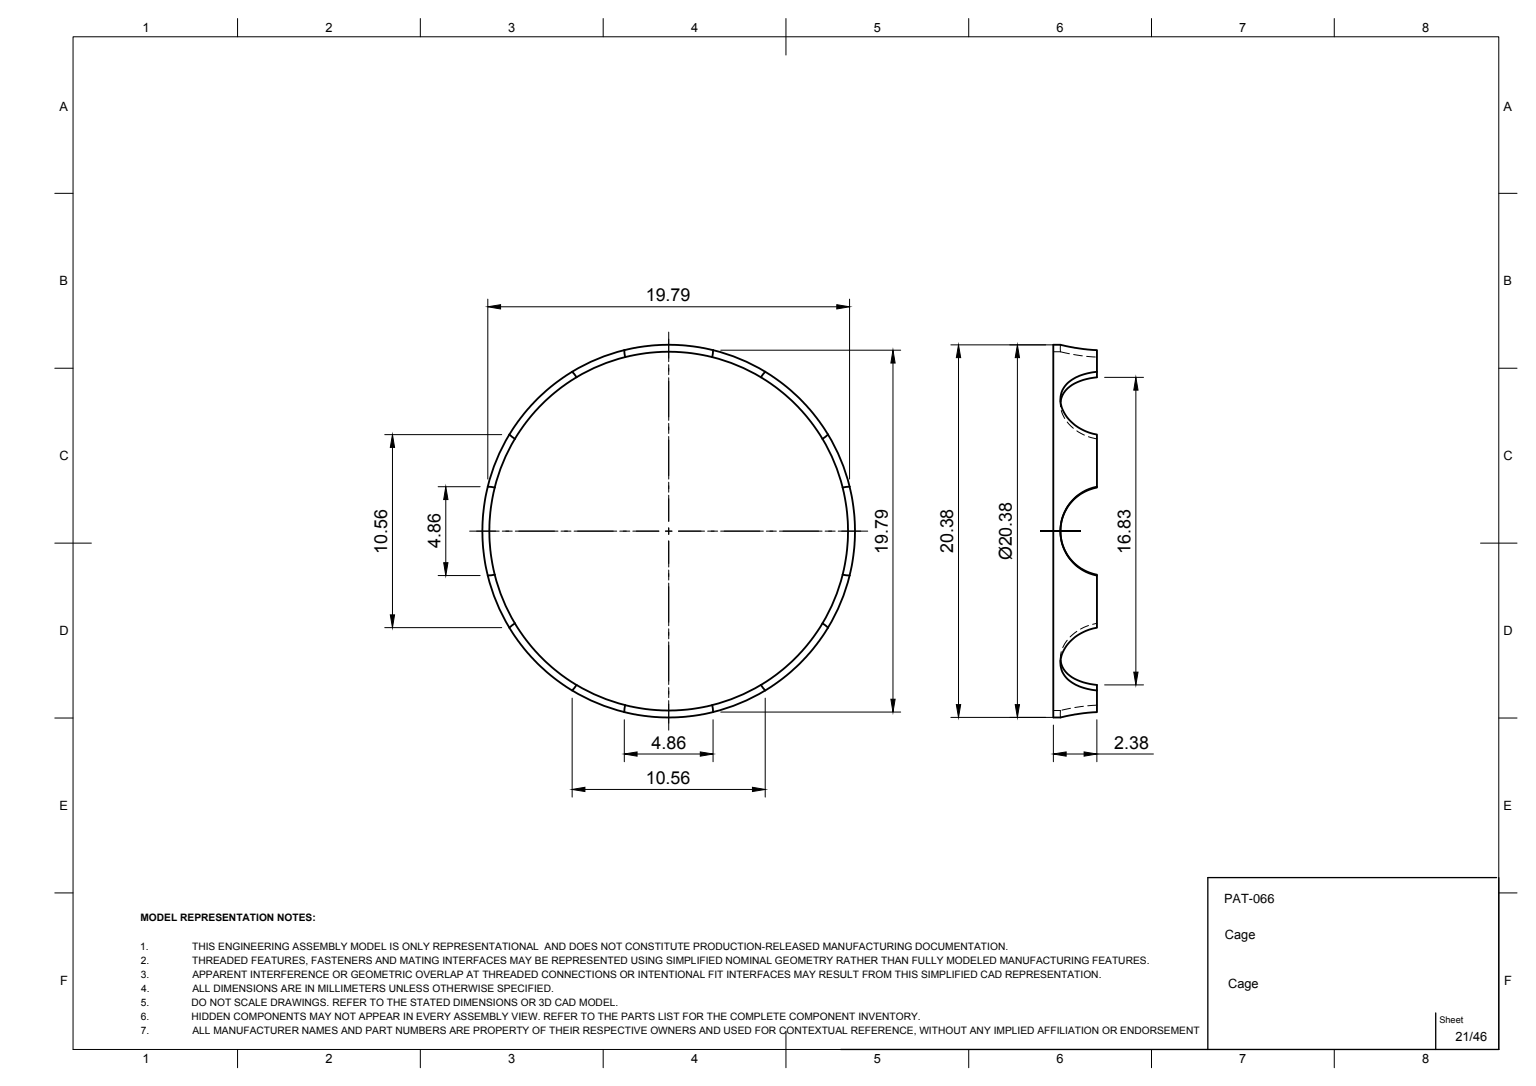
ISO-10303-21;
HEADER;
/* Generated by software containing ST-Developer
 * from STEP Tools, Inc. (www.steptools.com) 
 */

FILE_DESCRIPTION(
/* description */ ('Lever-operated bar clamp (toggle)'),
/* implementation_level */ '2;1');

FILE_NAME(
/* name */ 'Cage.step',
/* time_stamp */ '2026-10-28T03:25:02-07:00',
/* author */ (''),
/* organization */ (''),
/* preprocessor_version */ 'ST-DEVELOPER v20.2',
/* originating_system */ 'Autodesk Translation Framework v15.17.0.0',
/* authorisation */ '');

FILE_SCHEMA (('AUTOMOTIVE_DESIGN { 1 0 10303 214 3 1 1 }'));
ENDSEC;

DATA;
#10=MECHANICAL_DESIGN_GEOMETRIC_PRESENTATION_REPRESENTATION('',(#432),#12413);
#263=B_SPLINE_CURVE_WITH_KNOTS('',3,(#10837,#10838,#10839,#10840,#10841,
#10842,#10843,#10844,#10845,#10846,#10847,#10848,#10849,#10850,#10851,#10852,
#10853,#10854,#10855,#10856,#10857,#10858),.UNSPECIFIED.,.F.,.F.,(4,2,2,
2,2,2,2,2,2,2,4),(0.0473477652366656,0.126350602536658,0.189525903804987,
0.252701205073317,0.313298422430275,0.373895639787233,0.434492857144191,
0.495090074501149,0.558265375769478,0.621440677037807,0.7004435143378),
 .UNSPECIFIED.);
#264=B_SPLINE_CURVE_WITH_KNOTS('',3,(#10862,#10863,#10864,#10865,#10866,
#10867,#10868,#10869,#10870,#10871,#10872,#10873,#10874,#10875,#10876,#10877,
#10878,#10879,#10880,#10881,#10882,#10883),.UNSPECIFIED.,.F.,.F.,(4,2,2,
2,2,2,2,2,2,2,4),(0.0464897534940957,0.0852567806515119,0.170513561303024,
0.246687263103517,0.308657850341199,0.370628437578881,0.432599024816563,
0.494569612054245,0.570743313854739,0.656000094506251,0.694767121663666),
 .UNSPECIFIED.);
#265=B_SPLINE_CURVE_WITH_KNOTS('',3,(#10889,#10890,#10891,#10892,#10893,
#10894,#10895,#10896,#10897,#10898,#10899,#10900,#10901,#10902,#10903,#10904,
#10905,#10906,#10907,#10908,#10909,#10910),.UNSPECIFIED.,.F.,.F.,(4,2,2,
2,2,2,2,2,2,2,4),(0.0464897534940957,0.0852567806515118,0.170513561303024,
0.246687263103517,0.308657850341199,0.370628437578881,0.432599024816563,
0.494569612054245,0.570743313854738,0.65600009450625,0.694767121663666),
 .UNSPECIFIED.);
#266=B_SPLINE_CURVE_WITH_KNOTS('',3,(#10914,#10915,#10916,#10917,#10918,
#10919,#10920,#10921,#10922,#10923,#10924,#10925,#10926,#10927,#10928,#10929,
#10930,#10931,#10932,#10933,#10934,#10935),.UNSPECIFIED.,.F.,.F.,(4,2,2,
2,2,2,2,2,2,2,4),(0.0464897534940957,0.0852567806515119,0.170513561303024,
0.246687263103517,0.308657850341199,0.370628437578881,0.432599024816563,
0.494569612054245,0.570743313854739,0.656000094506251,0.694767121663666),
 .UNSPECIFIED.);
#267=B_SPLINE_CURVE_WITH_KNOTS('',3,(#10939,#10940,#10941,#10942,#10943,
#10944,#10945,#10946,#10947,#10948,#10949,#10950),.UNSPECIFIED.,.F.,.F.,
(4,2,2,2,2,4),(0.0464897534940957,0.0852567806515119,0.170513561303024,
0.246687263103517,0.308657850341199,0.370628437578881),.UNSPECIFIED.);
#268=B_SPLINE_CURVE_WITH_KNOTS('',3,(#10955,#10956,#10957,#10958,#10959,
#10960,#10961,#10962,#10963,#10964,#10965,#10966),.UNSPECIFIED.,.F.,.F.,
(4,2,2,2,2,4),(0.370628437578881,0.432599024816563,0.494569612054245,0.570743313854738,
0.65600009450625,0.694767121663666),.UNSPECIFIED.);
#269=B_SPLINE_CURVE_WITH_KNOTS('',3,(#10970,#10971,#10972,#10973,#10974,
#10975,#10976,#10977,#10978,#10979,#10980,#10981,#10982,#10983,#10984,#10985,
#10986,#10987,#10988,#10989,#10990,#10991),.UNSPECIFIED.,.F.,.F.,(4,2,2,
2,2,2,2,2,2,2,4),(0.0464897534940957,0.0852567806515121,0.170513561303024,
0.246687263103518,0.308657850341199,0.370628437578881,0.432599024816563,
0.494569612054245,0.570743313854738,0.65600009450625,0.694767121663666),
 .UNSPECIFIED.);
#270=B_SPLINE_CURVE_WITH_KNOTS('',3,(#10995,#10996,#10997,#10998,#10999,
#11000,#11001,#11002,#11003,#11004,#11005,#11006,#11007,#11008,#11009,#11010,
#11011,#11012,#11013,#11014,#11015,#11016),.UNSPECIFIED.,.F.,.F.,(4,2,2,
2,2,2,2,2,2,2,4),(0.0464897534940957,0.0852567806515119,0.170513561303024,
0.246687263103517,0.308657850341199,0.370628437578881,0.432599024816563,
0.494569612054245,0.570743313854738,0.65600009450625,0.694767121663667),
 .UNSPECIFIED.);
#271=B_SPLINE_CURVE_WITH_KNOTS('',3,(#11020,#11021,#11022,#11023,#11024,
#11025,#11026,#11027,#11028,#11029,#11030,#11031,#11032,#11033,#11034,#11035,
#11036,#11037,#11038,#11039,#11040,#11041),.UNSPECIFIED.,.F.,.F.,(4,2,2,
2,2,2,2,2,2,2,4),(0.0464897534940957,0.0852567806515119,0.170513561303024,
0.246687263103517,0.308657850341199,0.370628437578881,0.432599024816563,
0.494569612054245,0.570743313854738,0.65600009450625,0.694767121663666),
 .UNSPECIFIED.);
#272=B_SPLINE_CURVE_WITH_KNOTS('',3,(#11045,#11046,#11047,#11048,#11049,
#11050,#11051,#11052,#11053,#11054,#11055,#11056,#11057,#11058,#11059,#11060,
#11061,#11062,#11063,#11064,#11065,#11066),.UNSPECIFIED.,.F.,.F.,(4,2,2,
2,2,2,2,2,2,2,4),(0.0464897534940957,0.0852567806515119,0.170513561303024,
0.246687263103517,0.308657850341199,0.370628437578881,0.432599024816563,
0.494569612054245,0.570743313854739,0.656000094506251,0.694767121663667),
 .UNSPECIFIED.);
#273=B_SPLINE_CURVE_WITH_KNOTS('',3,(#11074,#11075,#11076,#11077,#11078,
#11079,#11080,#11081,#11082,#11083,#11084,#11085,#11086,#11087,#11088,#11089,
#11090,#11091,#11092,#11093,#11094,#11095),.UNSPECIFIED.,.F.,.F.,(4,2,2,
2,2,2,2,2,2,2,4),(0.0473477652366656,0.126350602536658,0.189525903804987,
0.252701205073316,0.313298422430274,0.373895639787232,0.434492857144191,
0.495090074501149,0.558265375769478,0.621440677037807,0.7004435143378),
 .UNSPECIFIED.);
#274=B_SPLINE_CURVE_WITH_KNOTS('',3,(#11103,#11104,#11105,#11106,#11107,
#11108,#11109,#11110,#11111,#11112,#11113,#11114,#11115,#11116,#11117,#11118,
#11119,#11120,#11121,#11122,#11123,#11124),.UNSPECIFIED.,.F.,.F.,(4,2,2,
2,2,2,2,2,2,2,4),(0.0473477652366656,0.126350602536658,0.189525903804987,
0.252701205073317,0.313298422430275,0.373895639787233,0.434492857144191,
0.495090074501149,0.558265375769478,0.621440677037807,0.7004435143378),
 .UNSPECIFIED.);
#275=B_SPLINE_CURVE_WITH_KNOTS('',3,(#11133,#11134,#11135,#11136,#11137,
#11138,#11139,#11140,#11141,#11142,#11143,#11144),.UNSPECIFIED.,.F.,.F.,
(4,2,2,2,2,4),(0.0473477652366656,0.126350602536658,0.189525903804987,0.252701205073316,
0.313298422430275,0.373895639787233),.UNSPECIFIED.);
#276=B_SPLINE_CURVE_WITH_KNOTS('',3,(#11146,#11147,#11148,#11149,#11150,
#11151,#11152,#11153,#11154,#11155,#11156,#11157),.UNSPECIFIED.,.F.,.F.,
(4,2,2,2,2,4),(0.373895639787233,0.434492857144191,0.495090074501149,0.558265375769478,
0.621440677037807,0.7004435143378),.UNSPECIFIED.);
#277=B_SPLINE_CURVE_WITH_KNOTS('',3,(#11164,#11165,#11166,#11167,#11168,
#11169,#11170,#11171,#11172,#11173,#11174,#11175,#11176,#11177,#11178,#11179,
#11180,#11181,#11182,#11183,#11184,#11185),.UNSPECIFIED.,.F.,.F.,(4,2,2,
2,2,2,2,2,2,2,4),(0.0473477652366656,0.126350602536658,0.189525903804987,
0.252701205073316,0.313298422430275,0.373895639787233,0.434492857144191,
0.495090074501149,0.558265375769478,0.621440677037807,0.7004435143378),
 .UNSPECIFIED.);
#278=B_SPLINE_CURVE_WITH_KNOTS('',3,(#11193,#11194,#11195,#11196,#11197,
#11198,#11199,#11200,#11201,#11202,#11203,#11204,#11205,#11206,#11207,#11208,
#11209,#11210,#11211,#11212,#11213,#11214),.UNSPECIFIED.,.F.,.F.,(4,2,2,
2,2,2,2,2,2,2,4),(0.0473477652366656,0.126350602536658,0.189525903804987,
0.252701205073317,0.313298422430275,0.373895639787233,0.434492857144191,
0.495090074501149,0.558265375769478,0.621440677037807,0.7004435143378),
 .UNSPECIFIED.);
#279=B_SPLINE_CURVE_WITH_KNOTS('',3,(#11222,#11223,#11224,#11225,#11226,
#11227,#11228,#11229,#11230,#11231,#11232,#11233,#11234,#11235,#11236,#11237,
#11238,#11239,#11240,#11241,#11242,#11243),.UNSPECIFIED.,.F.,.F.,(4,2,2,
2,2,2,2,2,2,2,4),(0.0473477652366656,0.126350602536658,0.189525903804987,
0.252701205073316,0.313298422430275,0.373895639787233,0.434492857144191,
0.495090074501149,0.558265375769478,0.621440677037807,0.7004435143378),
 .UNSPECIFIED.);
#280=B_SPLINE_CURVE_WITH_KNOTS('',3,(#11252,#11253,#11254,#11255,#11256,
#11257,#11258,#11259,#11260,#11261,#11262,#11263,#11264,#11265,#11266,#11267,
#11268,#11269,#11270,#11271,#11272,#11273),.UNSPECIFIED.,.F.,.F.,(4,2,2,
2,2,2,2,2,2,2,4),(0.0473477652366656,0.126350602536658,0.189525903804987,
0.252701205073317,0.313298422430275,0.373895639787233,0.434492857144191,
0.495090074501149,0.558265375769478,0.621440677037807,0.7004435143378),
 .UNSPECIFIED.);
#295=SPHERICAL_SURFACE('',#7386,0.247676);
#296=SPHERICAL_SURFACE('',#7402,0.247676);
#297=SPHERICAL_SURFACE('',#7407,0.247676);
#298=SPHERICAL_SURFACE('',#7412,0.247676);
#299=SPHERICAL_SURFACE('',#7417,0.247676);
#300=SPHERICAL_SURFACE('',#7422,0.247676);
#301=SPHERICAL_SURFACE('',#7427,0.247676);
#302=SPHERICAL_SURFACE('',#7435,0.247676);
#349=SHAPE_REPRESENTATION_RELATIONSHIP('SRR','None',#12589,#387);
#387=ADVANCED_BREP_SHAPE_REPRESENTATION('',(#478),#12386);
#432=STYLED_ITEM('',(#12869),#478);
#478=MANIFOLD_SOLID_BREP('Continuous crown cage',#6592);
#592=FACE_BOUND('',#1579,.T.);
#743=PLANE('',#7399);
#744=PLANE('',#7404);
#745=PLANE('',#7409);
#746=PLANE('',#7414);
#747=PLANE('',#7419);
#748=PLANE('',#7424);
#749=PLANE('',#7433);
#750=PLANE('',#7437);
#751=PLANE('',#7438);
#1063=FACE_OUTER_BOUND('',#1561,.T.);
#1064=FACE_OUTER_BOUND('',#1562,.T.);
#1065=FACE_OUTER_BOUND('',#1563,.T.);
#1066=FACE_OUTER_BOUND('',#1564,.T.);
#1067=FACE_OUTER_BOUND('',#1565,.T.);
#1068=FACE_OUTER_BOUND('',#1566,.T.);
#1069=FACE_OUTER_BOUND('',#1567,.T.);
#1070=FACE_OUTER_BOUND('',#1568,.T.);
#1071=FACE_OUTER_BOUND('',#1569,.T.);
#1072=FACE_OUTER_BOUND('',#1570,.T.);
#1073=FACE_OUTER_BOUND('',#1571,.T.);
#1074=FACE_OUTER_BOUND('',#1572,.T.);
#1075=FACE_OUTER_BOUND('',#1573,.T.);
#1076=FACE_OUTER_BOUND('',#1574,.T.);
#1077=FACE_OUTER_BOUND('',#1575,.T.);
#1078=FACE_OUTER_BOUND('',#1576,.T.);
#1079=FACE_OUTER_BOUND('',#1577,.T.);
#1080=FACE_OUTER_BOUND('',#1578,.T.);
#1081=FACE_OUTER_BOUND('',#1580,.T.);
#1561=EDGE_LOOP('',(#5125,#5126,#5127,#5128));
#1562=EDGE_LOOP('',(#5129,#5130,#5131,#5132,#5133,#5134,#5135,#5136,#5137,
#5138,#5139,#5140,#5141,#5142,#5143,#5144,#5145,#5146,#5147,#5148));
#1563=EDGE_LOOP('',(#5149,#5150,#5151,#5152));
#1564=EDGE_LOOP('',(#5153,#5154,#5155,#5156));
#1565=EDGE_LOOP('',(#5157,#5158,#5159,#5160));
#1566=EDGE_LOOP('',(#5161,#5162,#5163,#5164));
#1567=EDGE_LOOP('',(#5165,#5166,#5167,#5168));
#1568=EDGE_LOOP('',(#5169,#5170,#5171,#5172,#5173,#5174));
#1569=EDGE_LOOP('',(#5175,#5176,#5177,#5178));
#1570=EDGE_LOOP('',(#5179,#5180,#5181,#5182));
#1571=EDGE_LOOP('',(#5183,#5184,#5185,#5186));
#1572=EDGE_LOOP('',(#5187,#5188,#5189,#5190));
#1573=EDGE_LOOP('',(#5191,#5192,#5193,#5194));
#1574=EDGE_LOOP('',(#5195,#5196,#5197,#5198));
#1575=EDGE_LOOP('',(#5199,#5200,#5201,#5202,#5203,#5204,#5205,#5206,#5207,
#5208,#5209,#5210,#5211,#5212,#5213,#5214,#5215,#5216,#5217,#5218));
#1576=EDGE_LOOP('',(#5219,#5220,#5221,#5222));
#1577=EDGE_LOOP('',(#5223,#5224,#5225,#5226));
#1578=EDGE_LOOP('',(#5227));
#1579=EDGE_LOOP('',(#5228));
#1580=EDGE_LOOP('',(#5229,#5230,#5231,#5232));
#2050=LINE('',#10952,#2491);
#2051=LINE('',#11248,#2492);
#2491=VECTOR('',#8801,1.019052);
#2492=VECTOR('',#8878,0.980948);
#2886=CIRCLE('',#7387,0.243053047864041);
#2887=CIRCLE('',#7388,0.243053047864041);
#2888=CIRCLE('',#7390,1.019052);
#2889=CIRCLE('',#7391,1.019052);
#2890=CIRCLE('',#7392,1.019052);
#2891=CIRCLE('',#7393,1.019052);
#2892=CIRCLE('',#7394,1.019052);
#2893=CIRCLE('',#7395,1.019052);
#2894=CIRCLE('',#7396,1.019052);
#2895=CIRCLE('',#7397,1.019052);
#2896=CIRCLE('',#7398,1.019052);
#2897=CIRCLE('',#7400,0.980948);
#2898=CIRCLE('',#7401,0.243053047864041);
#2899=CIRCLE('',#7403,0.243053047864041);
#2900=CIRCLE('',#7405,0.980948);
#2901=CIRCLE('',#7406,0.243053047864041);
#2902=CIRCLE('',#7408,0.243053047864041);
#2903=CIRCLE('',#7410,0.980948);
#2904=CIRCLE('',#7411,0.243053047864041);
#2905=CIRCLE('',#7413,0.243053047864041);
#2906=CIRCLE('',#7415,0.980948);
#2907=CIRCLE('',#7416,0.243053047864041);
#2908=CIRCLE('',#7418,0.243053047864041);
#2909=CIRCLE('',#7420,0.980948);
#2910=CIRCLE('',#7421,0.243053047864041);
#2911=CIRCLE('',#7423,0.243053047864041);
#2912=CIRCLE('',#7425,0.980948);
#2913=CIRCLE('',#7426,0.243053047864041);
#2914=CIRCLE('',#7428,0.243053047864041);
#2915=CIRCLE('',#7430,0.980948);
#2916=CIRCLE('',#7431,0.980948);
#2917=CIRCLE('',#7432,0.980948);
#2918=CIRCLE('',#7434,0.243053047864041);
#2919=CIRCLE('',#7436,0.243053047864041);
#3317=VERTEX_POINT('',#10835);
#3318=VERTEX_POINT('',#10836);
#3319=VERTEX_POINT('',#10859);
#3320=VERTEX_POINT('',#10861);
#3321=VERTEX_POINT('',#10886);
#3322=VERTEX_POINT('',#10888);
#3323=VERTEX_POINT('',#10911);
#3324=VERTEX_POINT('',#10913);
#3325=VERTEX_POINT('',#10936);
#3326=VERTEX_POINT('',#10938);
#3327=VERTEX_POINT('',#10951);
#3328=VERTEX_POINT('',#10954);
#3329=VERTEX_POINT('',#10967);
#3330=VERTEX_POINT('',#10969);
#3331=VERTEX_POINT('',#10992);
#3332=VERTEX_POINT('',#10994);
#3333=VERTEX_POINT('',#11017);
#3334=VERTEX_POINT('',#11019);
#3335=VERTEX_POINT('',#11042);
#3336=VERTEX_POINT('',#11044);
#3337=VERTEX_POINT('',#11069);
#3338=VERTEX_POINT('',#11073);
#3339=VERTEX_POINT('',#11098);
#3340=VERTEX_POINT('',#11102);
#3341=VERTEX_POINT('',#11127);
#3342=VERTEX_POINT('',#11131);
#3343=VERTEX_POINT('',#11132);
#3344=VERTEX_POINT('',#11159);
#3345=VERTEX_POINT('',#11163);
#3346=VERTEX_POINT('',#11188);
#3347=VERTEX_POINT('',#11192);
#3348=VERTEX_POINT('',#11217);
#3349=VERTEX_POINT('',#11221);
#3350=VERTEX_POINT('',#11246);
#3351=VERTEX_POINT('',#11249);
#3352=VERTEX_POINT('',#11251);
#3967=EDGE_CURVE('',#3317,#3318,#263,.T.);
#3968=EDGE_CURVE('',#3319,#3317,#2886,.T.);
#3969=EDGE_CURVE('',#3320,#3319,#264,.T.);
#3970=EDGE_CURVE('',#3318,#3320,#2887,.T.);
#3971=EDGE_CURVE('',#3321,#3319,#2888,.T.);
#3972=EDGE_CURVE('',#3321,#3322,#265,.T.);
#3973=EDGE_CURVE('',#3323,#3322,#2889,.T.);
#3974=EDGE_CURVE('',#3323,#3324,#266,.T.);
#3975=EDGE_CURVE('',#3325,#3324,#2890,.T.);
#3976=EDGE_CURVE('',#3325,#3326,#267,.T.);
#3977=EDGE_CURVE('',#3326,#3327,#2050,.T.);
#3978=EDGE_CURVE('',#3327,#3327,#2891,.T.);
#3979=EDGE_CURVE('',#3326,#3328,#268,.T.);
#3980=EDGE_CURVE('',#3329,#3328,#2892,.T.);
#3981=EDGE_CURVE('',#3329,#3330,#269,.T.);
#3982=EDGE_CURVE('',#3331,#3330,#2893,.T.);
#3983=EDGE_CURVE('',#3331,#3332,#270,.T.);
#3984=EDGE_CURVE('',#3333,#3332,#2894,.T.);
#3985=EDGE_CURVE('',#3333,#3334,#271,.T.);
#3986=EDGE_CURVE('',#3335,#3334,#2895,.T.);
#3987=EDGE_CURVE('',#3335,#3336,#272,.T.);
#3988=EDGE_CURVE('',#3320,#3336,#2896,.T.);
#3989=EDGE_CURVE('',#3317,#3337,#2897,.T.);
#3990=EDGE_CURVE('',#3337,#3321,#2898,.T.);
#3991=EDGE_CURVE('',#3338,#3337,#273,.T.);
#3992=EDGE_CURVE('',#3322,#3338,#2899,.T.);
#3993=EDGE_CURVE('',#3338,#3339,#2900,.T.);
#3994=EDGE_CURVE('',#3339,#3323,#2901,.T.);
#3995=EDGE_CURVE('',#3340,#3339,#274,.T.);
#3996=EDGE_CURVE('',#3324,#3340,#2902,.T.);
#3997=EDGE_CURVE('',#3340,#3341,#2903,.T.);
#3998=EDGE_CURVE('',#3341,#3325,#2904,.T.);
#3999=EDGE_CURVE('',#3342,#3343,#275,.T.);
#4000=EDGE_CURVE('',#3328,#3342,#2905,.T.);
#4001=EDGE_CURVE('',#3343,#3341,#276,.T.);
#4002=EDGE_CURVE('',#3342,#3344,#2906,.T.);
#4003=EDGE_CURVE('',#3344,#3329,#2907,.T.);
#4004=EDGE_CURVE('',#3345,#3344,#277,.T.);
#4005=EDGE_CURVE('',#3330,#3345,#2908,.T.);
#4006=EDGE_CURVE('',#3345,#3346,#2909,.T.);
#4007=EDGE_CURVE('',#3346,#3331,#2910,.T.);
#4008=EDGE_CURVE('',#3347,#3346,#278,.T.);
#4009=EDGE_CURVE('',#3332,#3347,#2911,.T.);
#4010=EDGE_CURVE('',#3347,#3348,#2912,.T.);
#4011=EDGE_CURVE('',#3348,#3333,#2913,.T.);
#4012=EDGE_CURVE('',#3349,#3348,#279,.T.);
#4013=EDGE_CURVE('',#3334,#3349,#2914,.T.);
#4014=EDGE_CURVE('',#3350,#3350,#2915,.T.);
#4015=EDGE_CURVE('',#3350,#3343,#2051,.T.);
#4016=EDGE_CURVE('',#3351,#3318,#2916,.T.);
#4017=EDGE_CURVE('',#3351,#3352,#280,.T.);
#4018=EDGE_CURVE('',#3349,#3352,#2917,.T.);
#4019=EDGE_CURVE('',#3336,#3351,#2918,.T.);
#4020=EDGE_CURVE('',#3352,#3335,#2919,.T.);
#5125=ORIENTED_EDGE('',*,*,#3967,.F.);
#5126=ORIENTED_EDGE('',*,*,#3968,.F.);
#5127=ORIENTED_EDGE('',*,*,#3969,.F.);
#5128=ORIENTED_EDGE('',*,*,#3970,.F.);
#5129=ORIENTED_EDGE('',*,*,#3969,.T.);
#5130=ORIENTED_EDGE('',*,*,#3971,.F.);
#5131=ORIENTED_EDGE('',*,*,#3972,.T.);
#5132=ORIENTED_EDGE('',*,*,#3973,.F.);
#5133=ORIENTED_EDGE('',*,*,#3974,.T.);
#5134=ORIENTED_EDGE('',*,*,#3975,.F.);
#5135=ORIENTED_EDGE('',*,*,#3976,.T.);
#5136=ORIENTED_EDGE('',*,*,#3977,.T.);
#5137=ORIENTED_EDGE('',*,*,#3978,.F.);
#5138=ORIENTED_EDGE('',*,*,#3977,.F.);
#5139=ORIENTED_EDGE('',*,*,#3979,.T.);
#5140=ORIENTED_EDGE('',*,*,#3980,.F.);
#5141=ORIENTED_EDGE('',*,*,#3981,.T.);
#5142=ORIENTED_EDGE('',*,*,#3982,.F.);
#5143=ORIENTED_EDGE('',*,*,#3983,.T.);
#5144=ORIENTED_EDGE('',*,*,#3984,.F.);
#5145=ORIENTED_EDGE('',*,*,#3985,.T.);
#5146=ORIENTED_EDGE('',*,*,#3986,.F.);
#5147=ORIENTED_EDGE('',*,*,#3987,.T.);
#5148=ORIENTED_EDGE('',*,*,#3988,.F.);
#5149=ORIENTED_EDGE('',*,*,#3968,.T.);
#5150=ORIENTED_EDGE('',*,*,#3989,.T.);
#5151=ORIENTED_EDGE('',*,*,#3990,.T.);
#5152=ORIENTED_EDGE('',*,*,#3971,.T.);
#5153=ORIENTED_EDGE('',*,*,#3991,.F.);
#5154=ORIENTED_EDGE('',*,*,#3992,.F.);
#5155=ORIENTED_EDGE('',*,*,#3972,.F.);
#5156=ORIENTED_EDGE('',*,*,#3990,.F.);
#5157=ORIENTED_EDGE('',*,*,#3992,.T.);
#5158=ORIENTED_EDGE('',*,*,#3993,.T.);
#5159=ORIENTED_EDGE('',*,*,#3994,.T.);
#5160=ORIENTED_EDGE('',*,*,#3973,.T.);
#5161=ORIENTED_EDGE('',*,*,#3995,.F.);
#5162=ORIENTED_EDGE('',*,*,#3996,.F.);
#5163=ORIENTED_EDGE('',*,*,#3974,.F.);
#5164=ORIENTED_EDGE('',*,*,#3994,.F.);
#5165=ORIENTED_EDGE('',*,*,#3996,.T.);
#5166=ORIENTED_EDGE('',*,*,#3997,.T.);
#5167=ORIENTED_EDGE('',*,*,#3998,.T.);
#5168=ORIENTED_EDGE('',*,*,#3975,.T.);
#5169=ORIENTED_EDGE('',*,*,#3999,.F.);
#5170=ORIENTED_EDGE('',*,*,#4000,.F.);
#5171=ORIENTED_EDGE('',*,*,#3979,.F.);
#5172=ORIENTED_EDGE('',*,*,#3976,.F.);
#5173=ORIENTED_EDGE('',*,*,#3998,.F.);
#5174=ORIENTED_EDGE('',*,*,#4001,.F.);
#5175=ORIENTED_EDGE('',*,*,#4000,.T.);
#5176=ORIENTED_EDGE('',*,*,#4002,.T.);
#5177=ORIENTED_EDGE('',*,*,#4003,.T.);
#5178=ORIENTED_EDGE('',*,*,#3980,.T.);
#5179=ORIENTED_EDGE('',*,*,#4004,.F.);
#5180=ORIENTED_EDGE('',*,*,#4005,.F.);
#5181=ORIENTED_EDGE('',*,*,#3981,.F.);
#5182=ORIENTED_EDGE('',*,*,#4003,.F.);
#5183=ORIENTED_EDGE('',*,*,#4005,.T.);
#5184=ORIENTED_EDGE('',*,*,#4006,.T.);
#5185=ORIENTED_EDGE('',*,*,#4007,.T.);
#5186=ORIENTED_EDGE('',*,*,#3982,.T.);
#5187=ORIENTED_EDGE('',*,*,#4008,.F.);
#5188=ORIENTED_EDGE('',*,*,#4009,.F.);
#5189=ORIENTED_EDGE('',*,*,#3983,.F.);
#5190=ORIENTED_EDGE('',*,*,#4007,.F.);
#5191=ORIENTED_EDGE('',*,*,#4009,.T.);
#5192=ORIENTED_EDGE('',*,*,#4010,.T.);
#5193=ORIENTED_EDGE('',*,*,#4011,.T.);
#5194=ORIENTED_EDGE('',*,*,#3984,.T.);
#5195=ORIENTED_EDGE('',*,*,#3985,.F.);
#5196=ORIENTED_EDGE('',*,*,#4011,.F.);
#5197=ORIENTED_EDGE('',*,*,#4012,.F.);
#5198=ORIENTED_EDGE('',*,*,#4013,.F.);
#5199=ORIENTED_EDGE('',*,*,#4014,.F.);
#5200=ORIENTED_EDGE('',*,*,#4015,.T.);
#5201=ORIENTED_EDGE('',*,*,#4001,.T.);
#5202=ORIENTED_EDGE('',*,*,#3997,.F.);
#5203=ORIENTED_EDGE('',*,*,#3995,.T.);
#5204=ORIENTED_EDGE('',*,*,#3993,.F.);
#5205=ORIENTED_EDGE('',*,*,#3991,.T.);
#5206=ORIENTED_EDGE('',*,*,#3989,.F.);
#5207=ORIENTED_EDGE('',*,*,#3967,.T.);
#5208=ORIENTED_EDGE('',*,*,#4016,.F.);
#5209=ORIENTED_EDGE('',*,*,#4017,.T.);
#5210=ORIENTED_EDGE('',*,*,#4018,.F.);
#5211=ORIENTED_EDGE('',*,*,#4012,.T.);
#5212=ORIENTED_EDGE('',*,*,#4010,.F.);
#5213=ORIENTED_EDGE('',*,*,#4008,.T.);
#5214=ORIENTED_EDGE('',*,*,#4006,.F.);
#5215=ORIENTED_EDGE('',*,*,#4004,.T.);
#5216=ORIENTED_EDGE('',*,*,#4002,.F.);
#5217=ORIENTED_EDGE('',*,*,#3999,.T.);
#5218=ORIENTED_EDGE('',*,*,#4015,.F.);
#5219=ORIENTED_EDGE('',*,*,#3970,.T.);
#5220=ORIENTED_EDGE('',*,*,#3988,.T.);
#5221=ORIENTED_EDGE('',*,*,#4019,.T.);
#5222=ORIENTED_EDGE('',*,*,#4016,.T.);
#5223=ORIENTED_EDGE('',*,*,#3987,.F.);
#5224=ORIENTED_EDGE('',*,*,#4020,.F.);
#5225=ORIENTED_EDGE('',*,*,#4017,.F.);
#5226=ORIENTED_EDGE('',*,*,#4019,.F.);
#5227=ORIENTED_EDGE('',*,*,#3978,.T.);
#5228=ORIENTED_EDGE('',*,*,#4014,.T.);
#5229=ORIENTED_EDGE('',*,*,#4013,.T.);
#5230=ORIENTED_EDGE('',*,*,#4018,.T.);
#5231=ORIENTED_EDGE('',*,*,#4020,.T.);
#5232=ORIENTED_EDGE('',*,*,#3986,.T.);
#6099=CYLINDRICAL_SURFACE('',#7389,1.019052);
#6100=CYLINDRICAL_SURFACE('',#7429,0.980948);
#6338=ADVANCED_FACE('',(#1063),#295,.F.);
#6339=ADVANCED_FACE('',(#1064),#6099,.T.);
#6340=ADVANCED_FACE('',(#1065),#743,.T.);
#6341=ADVANCED_FACE('',(#1066),#296,.F.);
#6342=ADVANCED_FACE('',(#1067),#744,.T.);
#6343=ADVANCED_FACE('',(#1068),#297,.F.);
#6344=ADVANCED_FACE('',(#1069),#745,.T.);
#6345=ADVANCED_FACE('',(#1070),#298,.F.);
#6346=ADVANCED_FACE('',(#1071),#746,.T.);
#6347=ADVANCED_FACE('',(#1072),#299,.F.);
#6348=ADVANCED_FACE('',(#1073),#747,.T.);
#6349=ADVANCED_FACE('',(#1074),#300,.F.);
#6350=ADVANCED_FACE('',(#1075),#748,.T.);
#6351=ADVANCED_FACE('',(#1076),#301,.F.);
#6352=ADVANCED_FACE('',(#1077),#6100,.F.);
#6353=ADVANCED_FACE('',(#1078),#749,.T.);
#6354=ADVANCED_FACE('',(#1079),#302,.F.);
#6355=ADVANCED_FACE('',(#1080,#592),#750,.T.);
#6356=ADVANCED_FACE('',(#1081),#751,.T.);
#6592=CLOSED_SHELL('',(#6338,#6339,#6340,#6341,#6342,#6343,#6344,#6345,
#6346,#6347,#6348,#6349,#6350,#6351,#6352,#6353,#6354,#6355,#6356));
#7385=AXIS2_PLACEMENT_3D('',#10833,#8785,#8786);
#7386=AXIS2_PLACEMENT_3D('',#10834,#8787,#8788);
#7387=AXIS2_PLACEMENT_3D('',#10860,#8789,#8790);
#7388=AXIS2_PLACEMENT_3D('',#10884,#8791,#8792);
#7389=AXIS2_PLACEMENT_3D('',#10885,#8793,#8794);
#7390=AXIS2_PLACEMENT_3D('',#10887,#8795,#8796);
#7391=AXIS2_PLACEMENT_3D('',#10912,#8797,#8798);
#7392=AXIS2_PLACEMENT_3D('',#10937,#8799,#8800);
#7393=AXIS2_PLACEMENT_3D('',#10953,#8802,#8803);
#7394=AXIS2_PLACEMENT_3D('',#10968,#8804,#8805);
#7395=AXIS2_PLACEMENT_3D('',#10993,#8806,#8807);
#7396=AXIS2_PLACEMENT_3D('',#11018,#8808,#8809);
#7397=AXIS2_PLACEMENT_3D('',#11043,#8810,#8811);
#7398=AXIS2_PLACEMENT_3D('',#11067,#8812,#8813);
#7399=AXIS2_PLACEMENT_3D('',#11068,#8814,#8815);
#7400=AXIS2_PLACEMENT_3D('',#11070,#8816,#8817);
#7401=AXIS2_PLACEMENT_3D('',#11071,#8818,#8819);
#7402=AXIS2_PLACEMENT_3D('',#11072,#8820,#8821);
#7403=AXIS2_PLACEMENT_3D('',#11096,#8822,#8823);
#7404=AXIS2_PLACEMENT_3D('',#11097,#8824,#8825);
#7405=AXIS2_PLACEMENT_3D('',#11099,#8826,#8827);
#7406=AXIS2_PLACEMENT_3D('',#11100,#8828,#8829);
#7407=AXIS2_PLACEMENT_3D('',#11101,#8830,#8831);
#7408=AXIS2_PLACEMENT_3D('',#11125,#8832,#8833);
#7409=AXIS2_PLACEMENT_3D('',#11126,#8834,#8835);
#7410=AXIS2_PLACEMENT_3D('',#11128,#8836,#8837);
#7411=AXIS2_PLACEMENT_3D('',#11129,#8838,#8839);
#7412=AXIS2_PLACEMENT_3D('',#11130,#8840,#8841);
#7413=AXIS2_PLACEMENT_3D('',#11145,#8842,#8843);
#7414=AXIS2_PLACEMENT_3D('',#11158,#8844,#8845);
#7415=AXIS2_PLACEMENT_3D('',#11160,#8846,#8847);
#7416=AXIS2_PLACEMENT_3D('',#11161,#8848,#8849);
#7417=AXIS2_PLACEMENT_3D('',#11162,#8850,#8851);
#7418=AXIS2_PLACEMENT_3D('',#11186,#8852,#8853);
#7419=AXIS2_PLACEMENT_3D('',#11187,#8854,#8855);
#7420=AXIS2_PLACEMENT_3D('',#11189,#8856,#8857);
#7421=AXIS2_PLACEMENT_3D('',#11190,#8858,#8859);
#7422=AXIS2_PLACEMENT_3D('',#11191,#8860,#8861);
#7423=AXIS2_PLACEMENT_3D('',#11215,#8862,#8863);
#7424=AXIS2_PLACEMENT_3D('',#11216,#8864,#8865);
#7425=AXIS2_PLACEMENT_3D('',#11218,#8866,#8867);
#7426=AXIS2_PLACEMENT_3D('',#11219,#8868,#8869);
#7427=AXIS2_PLACEMENT_3D('',#11220,#8870,#8871);
#7428=AXIS2_PLACEMENT_3D('',#11244,#8872,#8873);
#7429=AXIS2_PLACEMENT_3D('',#11245,#8874,#8875);
#7430=AXIS2_PLACEMENT_3D('',#11247,#8876,#8877);
#7431=AXIS2_PLACEMENT_3D('',#11250,#8879,#8880);
#7432=AXIS2_PLACEMENT_3D('',#11274,#8881,#8882);
#7433=AXIS2_PLACEMENT_3D('',#11275,#8883,#8884);
#7434=AXIS2_PLACEMENT_3D('',#11276,#8885,#8886);
#7435=AXIS2_PLACEMENT_3D('',#11277,#8887,#8888);
#7436=AXIS2_PLACEMENT_3D('',#11278,#8889,#8890);
#7437=AXIS2_PLACEMENT_3D('',#11279,#8891,#8892);
#7438=AXIS2_PLACEMENT_3D('',#11280,#8893,#8894);
#8785=DIRECTION('axis',(0.,0.,1.));
#8786=DIRECTION('refdir',(1.,0.,0.));
#8787=DIRECTION('center_axis',(0.,0.,1.));
#8788=DIRECTION('ref_axis',(1.,0.,0.));
#8789=DIRECTION('center_axis',(0.,-1.,0.));
#8790=DIRECTION('ref_axis',(0.,0.,-1.));
#8791=DIRECTION('center_axis',(0.,-1.,0.));
#8792=DIRECTION('ref_axis',(0.,0.,-1.));
#8793=DIRECTION('center_axis',(0.,1.,0.));
#8794=DIRECTION('ref_axis',(1.,0.,0.));
#8795=DIRECTION('center_axis',(0.,1.,0.));
#8796=DIRECTION('ref_axis',(1.,0.,0.));
#8797=DIRECTION('center_axis',(0.,1.,0.));
#8798=DIRECTION('ref_axis',(1.,0.,0.));
#8799=DIRECTION('center_axis',(0.,1.,0.));
#8800=DIRECTION('ref_axis',(1.,0.,0.));
#8801=DIRECTION('',(0.,-1.,0.));
#8802=DIRECTION('center_axis',(0.,-1.,0.));
#8803=DIRECTION('ref_axis',(1.,0.,0.));
#8804=DIRECTION('center_axis',(0.,1.,0.));
#8805=DIRECTION('ref_axis',(1.,0.,0.));
#8806=DIRECTION('center_axis',(0.,1.,0.));
#8807=DIRECTION('ref_axis',(1.,0.,0.));
#8808=DIRECTION('center_axis',(0.,1.,0.));
#8809=DIRECTION('ref_axis',(1.,0.,0.));
#8810=DIRECTION('center_axis',(0.,1.,0.));
#8811=DIRECTION('ref_axis',(1.,0.,0.));
#8812=DIRECTION('center_axis',(0.,1.,0.));
#8813=DIRECTION('ref_axis',(1.,0.,0.));
#8814=DIRECTION('center_axis',(0.,1.,0.));
#8815=DIRECTION('ref_axis',(1.,0.,0.));
#8816=DIRECTION('center_axis',(0.,-1.,0.));
#8817=DIRECTION('ref_axis',(1.,0.,0.));
#8818=DIRECTION('center_axis',(0.,-1.,0.));
#8819=DIRECTION('ref_axis',(0.,0.,-1.));
#8820=DIRECTION('center_axis',(6.12323399573677E-17,0.,1.));
#8821=DIRECTION('ref_axis',(1.,0.,0.));
#8822=DIRECTION('center_axis',(0.,-1.,0.));
#8823=DIRECTION('ref_axis',(0.,0.,-1.));
#8824=DIRECTION('center_axis',(0.,1.,0.));
#8825=DIRECTION('ref_axis',(1.,0.,0.));
#8826=DIRECTION('center_axis',(0.,-1.,0.));
#8827=DIRECTION('ref_axis',(1.,0.,0.));
#8828=DIRECTION('center_axis',(0.,-1.,0.));
#8829=DIRECTION('ref_axis',(0.,0.,-1.));
#8830=DIRECTION('center_axis',(0.,0.,1.));
#8831=DIRECTION('ref_axis',(1.,0.,0.));
#8832=DIRECTION('center_axis',(0.,-1.,0.));
#8833=DIRECTION('ref_axis',(0.,0.,-1.));
#8834=DIRECTION('center_axis',(0.,1.,0.));
#8835=DIRECTION('ref_axis',(1.,0.,0.));
#8836=DIRECTION('center_axis',(0.,-1.,0.));
#8837=DIRECTION('ref_axis',(1.,0.,0.));
#8838=DIRECTION('center_axis',(0.,-1.,0.));
#8839=DIRECTION('ref_axis',(0.,0.,-1.));
#8840=DIRECTION('center_axis',(0.,0.,1.));
#8841=DIRECTION('ref_axis',(1.,0.,0.));
#8842=DIRECTION('center_axis',(0.,-1.,0.));
#8843=DIRECTION('ref_axis',(0.,0.,-1.));
#8844=DIRECTION('center_axis',(0.,1.,0.));
#8845=DIRECTION('ref_axis',(1.,0.,0.));
#8846=DIRECTION('center_axis',(0.,-1.,0.));
#8847=DIRECTION('ref_axis',(1.,0.,0.));
#8848=DIRECTION('center_axis',(0.,-1.,0.));
#8849=DIRECTION('ref_axis',(0.,0.,-1.));
#8850=DIRECTION('center_axis',(0.,0.,1.));
#8851=DIRECTION('ref_axis',(1.,0.,0.));
#8852=DIRECTION('center_axis',(0.,-1.,0.));
#8853=DIRECTION('ref_axis',(0.,0.,-1.));
#8854=DIRECTION('center_axis',(0.,1.,0.));
#8855=DIRECTION('ref_axis',(1.,0.,0.));
#8856=DIRECTION('center_axis',(0.,-1.,0.));
#8857=DIRECTION('ref_axis',(1.,0.,0.));
#8858=DIRECTION('center_axis',(0.,-1.,0.));
#8859=DIRECTION('ref_axis',(0.,0.,-1.));
#8860=DIRECTION('center_axis',(6.12323399573676E-17,0.,1.));
#8861=DIRECTION('ref_axis',(1.,0.,0.));
#8862=DIRECTION('center_axis',(0.,-1.,0.));
#8863=DIRECTION('ref_axis',(0.,0.,-1.));
#8864=DIRECTION('center_axis',(0.,1.,0.));
#8865=DIRECTION('ref_axis',(1.,0.,0.));
#8866=DIRECTION('center_axis',(0.,-1.,0.));
#8867=DIRECTION('ref_axis',(1.,0.,0.));
#8868=DIRECTION('center_axis',(0.,-1.,0.));
#8869=DIRECTION('ref_axis',(0.,0.,-1.));
#8870=DIRECTION('center_axis',(0.,0.,1.));
#8871=DIRECTION('ref_axis',(1.,0.,0.));
#8872=DIRECTION('center_axis',(0.,-1.,0.));
#8873=DIRECTION('ref_axis',(0.,0.,-1.));
#8874=DIRECTION('center_axis',(0.,1.,0.));
#8875=DIRECTION('ref_axis',(1.,0.,0.));
#8876=DIRECTION('center_axis',(0.,1.,0.));
#8877=DIRECTION('ref_axis',(1.,0.,0.));
#8878=DIRECTION('',(0.,1.,0.));
#8879=DIRECTION('center_axis',(0.,-1.,0.));
#8880=DIRECTION('ref_axis',(1.,0.,0.));
#8881=DIRECTION('center_axis',(0.,-1.,0.));
#8882=DIRECTION('ref_axis',(1.,0.,0.));
#8883=DIRECTION('center_axis',(0.,1.,0.));
#8884=DIRECTION('ref_axis',(1.,0.,0.));
#8885=DIRECTION('center_axis',(0.,-1.,0.));
#8886=DIRECTION('ref_axis',(0.,0.,-1.));
#8887=DIRECTION('center_axis',(0.,0.,1.));
#8888=DIRECTION('ref_axis',(1.,0.,0.));
#8889=DIRECTION('center_axis',(0.,-1.,0.));
#8890=DIRECTION('ref_axis',(0.,0.,-1.));
#8891=DIRECTION('center_axis',(0.,-1.,0.));
#8892=DIRECTION('ref_axis',(-1.,0.,0.));
#8893=DIRECTION('center_axis',(0.,1.,0.));
#8894=DIRECTION('ref_axis',(1.,0.,0.));
#10833=CARTESIAN_POINT('',(0.,0.,0.));
#10834=CARTESIAN_POINT('Origin',(0.707106781186547,0.,0.707106781186548));
#10835=CARTESIAN_POINT('',(0.504455939115715,-0.04763,0.841298510752802));
#10836=CARTESIAN_POINT('',(0.841298510752802,-0.04763,0.504455939115715));
#10837=CARTESIAN_POINT('Ctrl Pts',(0.504455939115715,-0.04763,0.841298510752802));
#10838=CARTESIAN_POINT('Ctrl Pts',(0.508899795931835,-0.0740444353928835,
0.838633903678357));
#10839=CARTESIAN_POINT('Ctrl Pts',(0.517157748491652,-0.0999305678883309,
0.833661031856294));
#10840=CARTESIAN_POINT('Ctrl Pts',(0.537715343527944,-0.142345102874864,
0.820511285096538));
#10841=CARTESIAN_POINT('Ctrl Pts',(0.548874290046456,-0.159766064500479,
0.813159949759));
#10842=CARTESIAN_POINT('Ctrl Pts',(0.573915184558107,-0.190326085855194,
0.795684265985089));
#10843=CARTESIAN_POINT('Ctrl Pts',(0.587792702767295,-0.203463743702801,
0.78555112003688));
#10844=CARTESIAN_POINT('Ctrl Pts',(0.615966552324775,-0.224161999508995,
0.763642258217233));
#10845=CARTESIAN_POINT('Ctrl Pts',(0.631684198665438,-0.232861760990032,
0.750785745543687));
#10846=CARTESIAN_POINT('Ctrl Pts',(0.663382628119203,-0.244251601209411,
0.722929908501543));
#10847=CARTESIAN_POINT('Ctrl Pts',(0.679352081686668,-0.246942143572133,
0.707917883896095));
#10848=CARTESIAN_POINT('Ctrl Pts',(0.707917883896095,-0.246942143572133,
0.679352081686668));
#10849=CARTESIAN_POINT('Ctrl Pts',(0.722929908501543,-0.244251601209411,
0.663382628119203));
#10850=CARTESIAN_POINT('Ctrl Pts',(0.750785745543687,-0.232861760990032,
0.631684198665439));
#10851=CARTESIAN_POINT('Ctrl Pts',(0.763642258217232,-0.224161999508995,
0.615966552324775));
#10852=CARTESIAN_POINT('Ctrl Pts',(0.78555112003688,-0.203463743702801,
0.587792702767295));
#10853=CARTESIAN_POINT('Ctrl Pts',(0.795684265985088,-0.190326085855194,
0.573915184558108));
#10854=CARTESIAN_POINT('Ctrl Pts',(0.813159949759,-0.15976606450048,0.548874290046456));
#10855=CARTESIAN_POINT('Ctrl Pts',(0.820511285096538,-0.142345102874864,
0.537715343527944));
#10856=CARTESIAN_POINT('Ctrl Pts',(0.833661031856294,-0.099930567888331,
0.517157748491653));
#10857=CARTESIAN_POINT('Ctrl Pts',(0.838633903678357,-0.0740444353928835,
0.508899795931835));
#10858=CARTESIAN_POINT('Ctrl Pts',(0.841298510752801,-0.0476299999999999,
0.504455939115715));
#10859=CARTESIAN_POINT('',(0.528110872004958,-0.04763,0.871530771444223));
#10860=CARTESIAN_POINT('Origin',(0.707106781186547,-0.04763,0.707106781186548));
#10861=CARTESIAN_POINT('',(0.871530771444223,-0.04763,0.528110872004959));
#10862=CARTESIAN_POINT('Ctrl Pts',(0.871530771444223,-0.0476300000000001,
0.528110872004958));
#10863=CARTESIAN_POINT('Ctrl Pts',(0.87014664509073,-0.0609922781173483,
0.530395067942936));
#10864=CARTESIAN_POINT('Ctrl Pts',(0.868149331745851,-0.0742967091364493,
0.533674141594226));
#10865=CARTESIAN_POINT('Ctrl Pts',(0.85981294420286,-0.115492077056649,
0.54708917182331));
#10866=CARTESIAN_POINT('Ctrl Pts',(0.850993704737257,-0.141695629206859,
0.560922177770136));
#10867=CARTESIAN_POINT('Ctrl Pts',(0.830754510485543,-0.181890537957859,
0.590422647829571));
#10868=CARTESIAN_POINT('Ctrl Pts',(0.816896541396381,-0.201072148666545,
0.609616703125488));
#10869=CARTESIAN_POINT('Ctrl Pts',(0.792310597819928,-0.223955109275652,
0.641117951819998));
#10870=CARTESIAN_POINT('Ctrl Pts',(0.779109323683612,-0.232742381310829,
0.657208095763053));
#10871=CARTESIAN_POINT('Ctrl Pts',(0.750552691816206,-0.244234834628584,
0.68964083160521));
#10872=CARTESIAN_POINT('Ctrl Pts',(0.735185187071673,-0.246942143572133,
0.705971972091755));
#10873=CARTESIAN_POINT('Ctrl Pts',(0.705971972091754,-0.246942143572133,
0.735185187071673));
#10874=CARTESIAN_POINT('Ctrl Pts',(0.689640831605209,-0.244234834628584,
0.750552691816206));
#10875=CARTESIAN_POINT('Ctrl Pts',(0.657208095763052,-0.232742381310829,
0.779109323683612));
#10876=CARTESIAN_POINT('Ctrl Pts',(0.641117951819998,-0.223955109275652,
0.792310597819928));
#10877=CARTESIAN_POINT('Ctrl Pts',(0.609616703125487,-0.201072148666545,
0.816896541396382));
#10878=CARTESIAN_POINT('Ctrl Pts',(0.590422647829571,-0.181890537957858,
0.830754510485544));
#10879=CARTESIAN_POINT('Ctrl Pts',(0.560922177770135,-0.141695629206858,
0.850993704737257));
#10880=CARTESIAN_POINT('Ctrl Pts',(0.547089171823309,-0.115492077056649,
0.859812944202861));
#10881=CARTESIAN_POINT('Ctrl Pts',(0.533674141594226,-0.0742967091364491,
0.868149331745852));
#10882=CARTESIAN_POINT('Ctrl Pts',(0.530395067942936,-0.0609922781173483,
0.870146645090731));
#10883=CARTESIAN_POINT('Ctrl Pts',(0.528110872004958,-0.0476300000000001,
0.871530771444223));
#10884=CARTESIAN_POINT('Origin',(0.707106781186547,-0.04763,0.707106781186548));
#10885=CARTESIAN_POINT('Origin',(0.,-0.166705,0.));
#10886=CARTESIAN_POINT('',(0.242834539687906,-0.04763,0.989696097314));
#10887=CARTESIAN_POINT('Origin',(0.,-0.04763,0.));
#10888=CARTESIAN_POINT('',(-0.242834539687907,-0.04763,0.989696097314));
#10889=CARTESIAN_POINT('Ctrl Pts',(0.242834539687906,-0.04763,0.989696097314));
#10890=CARTESIAN_POINT('Ctrl Pts',(0.24024064412003,-0.0609922781173483,
0.990332542620729));
#10891=CARTESIAN_POINT('Ctrl Pts',(0.236509675094874,-0.0742967091364492,
0.991238884025248));
#10892=CARTESIAN_POINT('Ctrl Pts',(0.221129100087819,-0.115492077056649,
0.994830026707808));
#10893=CARTESIAN_POINT('Ctrl Pts',(0.205111543747588,-0.141695629206859,
0.998375294985966));
#10894=CARTESIAN_POINT('Ctrl Pts',(0.169940289819232,-0.181890537957859,
1.00492400591205));
#10895=CARTESIAN_POINT('Ctrl Pts',(0.1465689792446,-0.201072148666545,1.00869718865384));
#10896=CARTESIAN_POINT('Ctrl Pts',(0.106909345252087,-0.223955109275652,
1.01358704779679));
#10897=CARTESIAN_POINT('Ctrl Pts',(0.0861971848975941,-0.232742381310829,
1.0156297872271));
#10898=CARTESIAN_POINT('Ctrl Pts',(0.0430711894098822,-0.244234834628584,
1.01837060663223));
#10899=CARTESIAN_POINT('Ctrl Pts',(0.0206568624125605,-0.246942143572133,
1.019052));
#10900=CARTESIAN_POINT('Ctrl Pts',(-0.0206568624125608,-0.246942143572133,
1.019052));
#10901=CARTESIAN_POINT('Ctrl Pts',(-0.0430711894098825,-0.244234834628584,
1.01837060663223));
#10902=CARTESIAN_POINT('Ctrl Pts',(-0.0861971848975943,-0.232742381310829,
1.0156297872271));
#10903=CARTESIAN_POINT('Ctrl Pts',(-0.106909345252088,-0.223955109275652,
1.01358704779679));
#10904=CARTESIAN_POINT('Ctrl Pts',(-0.1465689792446,-0.201072148666545,
1.00869718865384));
#10905=CARTESIAN_POINT('Ctrl Pts',(-0.169940289819232,-0.181890537957859,
1.00492400591205));
#10906=CARTESIAN_POINT('Ctrl Pts',(-0.205111543747588,-0.141695629206859,
0.998375294985966));
#10907=CARTESIAN_POINT('Ctrl Pts',(-0.221129100087819,-0.115492077056649,
0.994830026707808));
#10908=CARTESIAN_POINT('Ctrl Pts',(-0.236509675094875,-0.0742967091364493,
0.991238884025248));
#10909=CARTESIAN_POINT('Ctrl Pts',(-0.24024064412003,-0.0609922781173483,
0.990332542620729));
#10910=CARTESIAN_POINT('Ctrl Pts',(-0.242834539687907,-0.04763,0.989696097314));
#10911=CARTESIAN_POINT('',(-0.528110872004959,-0.04763,0.871530771444223));
#10912=CARTESIAN_POINT('Origin',(0.,-0.04763,0.));
#10913=CARTESIAN_POINT('',(-0.871530771444223,-0.04763,0.528110872004958));
#10914=CARTESIAN_POINT('Ctrl Pts',(-0.528110872004958,-0.0476300000000001,
0.871530771444223));
#10915=CARTESIAN_POINT('Ctrl Pts',(-0.530395067942936,-0.0609922781173484,
0.87014664509073));
#10916=CARTESIAN_POINT('Ctrl Pts',(-0.533674141594226,-0.0742967091364493,
0.868149331745851));
#10917=CARTESIAN_POINT('Ctrl Pts',(-0.54708917182331,-0.115492077056649,
0.85981294420286));
#10918=CARTESIAN_POINT('Ctrl Pts',(-0.560922177770136,-0.141695629206859,
0.850993704737257));
#10919=CARTESIAN_POINT('Ctrl Pts',(-0.590422647829571,-0.181890537957859,
0.830754510485543));
#10920=CARTESIAN_POINT('Ctrl Pts',(-0.609616703125488,-0.201072148666545,
0.816896541396381));
#10921=CARTESIAN_POINT('Ctrl Pts',(-0.641117951819998,-0.223955109275652,
0.792310597819928));
#10922=CARTESIAN_POINT('Ctrl Pts',(-0.657208095763053,-0.232742381310829,
0.779109323683611));
#10923=CARTESIAN_POINT('Ctrl Pts',(-0.68964083160521,-0.244234834628584,
0.750552691816205));
#10924=CARTESIAN_POINT('Ctrl Pts',(-0.705971972091755,-0.246942143572133,
0.735185187071673));
#10925=CARTESIAN_POINT('Ctrl Pts',(-0.735185187071673,-0.246942143572133,
0.705971972091754));
#10926=CARTESIAN_POINT('Ctrl Pts',(-0.750552691816206,-0.244234834628584,
0.689640831605209));
#10927=CARTESIAN_POINT('Ctrl Pts',(-0.779109323683612,-0.232742381310829,
0.657208095763052));
#10928=CARTESIAN_POINT('Ctrl Pts',(-0.792310597819928,-0.223955109275652,
0.641117951819998));
#10929=CARTESIAN_POINT('Ctrl Pts',(-0.816896541396382,-0.201072148666545,
0.609616703125487));
#10930=CARTESIAN_POINT('Ctrl Pts',(-0.830754510485544,-0.181890537957858,
0.590422647829571));
#10931=CARTESIAN_POINT('Ctrl Pts',(-0.850993704737257,-0.141695629206858,
0.560922177770135));
#10932=CARTESIAN_POINT('Ctrl Pts',(-0.859812944202861,-0.115492077056649,
0.547089171823309));
#10933=CARTESIAN_POINT('Ctrl Pts',(-0.868149331745852,-0.0742967091364491,
0.533674141594226));
#10934=CARTESIAN_POINT('Ctrl Pts',(-0.870146645090731,-0.0609922781173483,
0.530395067942936));
#10935=CARTESIAN_POINT('Ctrl Pts',(-0.871530771444223,-0.04763,0.528110872004958));
#10936=CARTESIAN_POINT('',(-0.989696097314,-0.04763,0.242834539687906));
#10937=CARTESIAN_POINT('Origin',(0.,-0.04763,0.));
#10938=CARTESIAN_POINT('',(-1.019052,-0.246942143572133,1.248489836334E-16));
#10939=CARTESIAN_POINT('Ctrl Pts',(-0.989696097314,-0.04763,0.242834539687906));
#10940=CARTESIAN_POINT('Ctrl Pts',(-0.990332542620729,-0.0609922781173483,
0.24024064412003));
#10941=CARTESIAN_POINT('Ctrl Pts',(-0.991238884025248,-0.0742967091364492,
0.236509675094874));
#10942=CARTESIAN_POINT('Ctrl Pts',(-0.994830026707808,-0.115492077056649,
0.221129100087819));
#10943=CARTESIAN_POINT('Ctrl Pts',(-0.998375294985966,-0.141695629206859,
0.205111543747588));
#10944=CARTESIAN_POINT('Ctrl Pts',(-1.00492400591205,-0.181890537957859,
0.169940289819232));
#10945=CARTESIAN_POINT('Ctrl Pts',(-1.00869718865384,-0.201072148666545,
0.1465689792446));
#10946=CARTESIAN_POINT('Ctrl Pts',(-1.01358704779679,-0.223955109275652,
0.106909345252088));
#10947=CARTESIAN_POINT('Ctrl Pts',(-1.0156297872271,-0.232742381310829,
0.0861971848975944));
#10948=CARTESIAN_POINT('Ctrl Pts',(-1.01837060663223,-0.244234834628584,
0.0430711894098825));
#10949=CARTESIAN_POINT('Ctrl Pts',(-1.019052,-0.246942143572133,0.0206568624125608));
#10950=CARTESIAN_POINT('Ctrl Pts',(-1.019052,-0.246942143572133,1.2490009027033E-16));
#10951=CARTESIAN_POINT('',(-1.019052,-0.28578,1.24797876996471E-16));
#10952=CARTESIAN_POINT('',(-1.019052,-0.166705,1.24797876996471E-16));
#10953=CARTESIAN_POINT('Origin',(0.,-0.28578,0.));
#10954=CARTESIAN_POINT('',(-0.989696097314,-0.04763,-0.242834539687906));
#10955=CARTESIAN_POINT('Ctrl Pts',(-1.019052,-0.246942143572133,1.2490009027033E-16));
#10956=CARTESIAN_POINT('Ctrl Pts',(-1.019052,-0.246942143572133,-0.0206568624125605));
#10957=CARTESIAN_POINT('Ctrl Pts',(-1.01837060663223,-0.244234834628584,
-0.0430711894098822));
#10958=CARTESIAN_POINT('Ctrl Pts',(-1.0156297872271,-0.232742381310829,
-0.0861971848975941));
#10959=CARTESIAN_POINT('Ctrl Pts',(-1.01358704779679,-0.223955109275652,
-0.106909345252087));
#10960=CARTESIAN_POINT('Ctrl Pts',(-1.00869718865384,-0.201072148666546,
-0.1465689792446));
#10961=CARTESIAN_POINT('Ctrl Pts',(-1.00492400591205,-0.181890537957859,
-0.169940289819232));
#10962=CARTESIAN_POINT('Ctrl Pts',(-0.998375294985966,-0.141695629206859,
-0.205111543747588));
#10963=CARTESIAN_POINT('Ctrl Pts',(-0.994830026707808,-0.11549207705665,
-0.221129100087819));
#10964=CARTESIAN_POINT('Ctrl Pts',(-0.991238884025248,-0.0742967091364495,
-0.236509675094874));
#10965=CARTESIAN_POINT('Ctrl Pts',(-0.990332542620729,-0.0609922781173484,
-0.24024064412003));
#10966=CARTESIAN_POINT('Ctrl Pts',(-0.989696097314,-0.0476300000000001,
-0.242834539687907));
#10967=CARTESIAN_POINT('',(-0.871530771444223,-0.04763,-0.528110872004958));
#10968=CARTESIAN_POINT('Origin',(0.,-0.04763,0.));
#10969=CARTESIAN_POINT('',(-0.528110872004958,-0.04763,-0.871530771444223));
#10970=CARTESIAN_POINT('Ctrl Pts',(-0.871530771444223,-0.0476300000000001,
-0.528110872004958));
#10971=CARTESIAN_POINT('Ctrl Pts',(-0.87014664509073,-0.0609922781173484,
-0.530395067942936));
#10972=CARTESIAN_POINT('Ctrl Pts',(-0.868149331745851,-0.0742967091364494,
-0.533674141594226));
#10973=CARTESIAN_POINT('Ctrl Pts',(-0.85981294420286,-0.115492077056649,
-0.54708917182331));
#10974=CARTESIAN_POINT('Ctrl Pts',(-0.850993704737257,-0.141695629206859,
-0.560922177770136));
#10975=CARTESIAN_POINT('Ctrl Pts',(-0.830754510485543,-0.181890537957859,
-0.590422647829571));
#10976=CARTESIAN_POINT('Ctrl Pts',(-0.816896541396381,-0.201072148666546,
-0.609616703125488));
#10977=CARTESIAN_POINT('Ctrl Pts',(-0.792310597819928,-0.223955109275652,
-0.641117951819999));
#10978=CARTESIAN_POINT('Ctrl Pts',(-0.779109323683611,-0.232742381310829,
-0.657208095763053));
#10979=CARTESIAN_POINT('Ctrl Pts',(-0.750552691816205,-0.244234834628584,
-0.68964083160521));
#10980=CARTESIAN_POINT('Ctrl Pts',(-0.735185187071673,-0.246942143572133,
-0.705971972091755));
#10981=CARTESIAN_POINT('Ctrl Pts',(-0.705971972091754,-0.246942143572133,
-0.735185187071673));
#10982=CARTESIAN_POINT('Ctrl Pts',(-0.68964083160521,-0.244234834628584,
-0.750552691816206));
#10983=CARTESIAN_POINT('Ctrl Pts',(-0.657208095763052,-0.232742381310829,
-0.779109323683612));
#10984=CARTESIAN_POINT('Ctrl Pts',(-0.641117951819998,-0.223955109275652,
-0.792310597819928));
#10985=CARTESIAN_POINT('Ctrl Pts',(-0.609616703125488,-0.201072148666545,
-0.816896541396381));
#10986=CARTESIAN_POINT('Ctrl Pts',(-0.590422647829571,-0.181890537957859,
-0.830754510485543));
#10987=CARTESIAN_POINT('Ctrl Pts',(-0.560922177770136,-0.141695629206859,
-0.850993704737257));
#10988=CARTESIAN_POINT('Ctrl Pts',(-0.54708917182331,-0.115492077056649,
-0.85981294420286));
#10989=CARTESIAN_POINT('Ctrl Pts',(-0.533674141594226,-0.0742967091364494,
-0.868149331745852));
#10990=CARTESIAN_POINT('Ctrl Pts',(-0.530395067942936,-0.0609922781173484,
-0.870146645090731));
#10991=CARTESIAN_POINT('Ctrl Pts',(-0.528110872004958,-0.0476300000000001,
-0.871530771444223));
#10992=CARTESIAN_POINT('',(-0.242834539687906,-0.04763,-0.989696097314));
#10993=CARTESIAN_POINT('Origin',(0.,-0.04763,0.));
#10994=CARTESIAN_POINT('',(0.242834539687906,-0.04763,-0.989696097314));
#10995=CARTESIAN_POINT('Ctrl Pts',(-0.242834539687907,-0.04763,-0.989696097314));
#10996=CARTESIAN_POINT('Ctrl Pts',(-0.24024064412003,-0.0609922781173483,
-0.990332542620729));
#10997=CARTESIAN_POINT('Ctrl Pts',(-0.236509675094874,-0.0742967091364493,
-0.991238884025248));
#10998=CARTESIAN_POINT('Ctrl Pts',(-0.221129100087819,-0.115492077056649,
-0.994830026707808));
#10999=CARTESIAN_POINT('Ctrl Pts',(-0.205111543747588,-0.141695629206859,
-0.998375294985966));
#11000=CARTESIAN_POINT('Ctrl Pts',(-0.169940289819232,-0.181890537957859,
-1.00492400591205));
#11001=CARTESIAN_POINT('Ctrl Pts',(-0.1465689792446,-0.201072148666545,
-1.00869718865384));
#11002=CARTESIAN_POINT('Ctrl Pts',(-0.106909345252087,-0.223955109275652,
-1.01358704779679));
#11003=CARTESIAN_POINT('Ctrl Pts',(-0.0861971848975942,-0.232742381310829,
-1.0156297872271));
#11004=CARTESIAN_POINT('Ctrl Pts',(-0.0430711894098823,-0.244234834628584,
-1.01837060663223));
#11005=CARTESIAN_POINT('Ctrl Pts',(-0.0206568624125606,-0.246942143572133,
-1.019052));
#11006=CARTESIAN_POINT('Ctrl Pts',(0.0206568624125607,-0.246942143572133,
-1.019052));
#11007=CARTESIAN_POINT('Ctrl Pts',(0.0430711894098824,-0.244234834628584,
-1.01837060663223));
#11008=CARTESIAN_POINT('Ctrl Pts',(0.0861971848975943,-0.232742381310829,
-1.0156297872271));
#11009=CARTESIAN_POINT('Ctrl Pts',(0.106909345252088,-0.223955109275652,
-1.01358704779679));
#11010=CARTESIAN_POINT('Ctrl Pts',(0.1465689792446,-0.201072148666545,-1.00869718865384));
#11011=CARTESIAN_POINT('Ctrl Pts',(0.169940289819232,-0.181890537957859,
-1.00492400591205));
#11012=CARTESIAN_POINT('Ctrl Pts',(0.205111543747588,-0.141695629206859,
-0.998375294985966));
#11013=CARTESIAN_POINT('Ctrl Pts',(0.221129100087819,-0.115492077056649,
-0.994830026707808));
#11014=CARTESIAN_POINT('Ctrl Pts',(0.236509675094874,-0.0742967091364493,
-0.991238884025248));
#11015=CARTESIAN_POINT('Ctrl Pts',(0.24024064412003,-0.0609922781173484,
-0.990332542620729));
#11016=CARTESIAN_POINT('Ctrl Pts',(0.242834539687907,-0.04763,-0.989696097314));
#11017=CARTESIAN_POINT('',(0.528110872004958,-0.04763,-0.871530771444223));
#11018=CARTESIAN_POINT('Origin',(0.,-0.04763,0.));
#11019=CARTESIAN_POINT('',(0.871530771444223,-0.04763,-0.528110872004958));
#11020=CARTESIAN_POINT('Ctrl Pts',(0.528110872004958,-0.0476300000000001,
-0.871530771444223));
#11021=CARTESIAN_POINT('Ctrl Pts',(0.530395067942936,-0.0609922781173484,
-0.870146645090731));
#11022=CARTESIAN_POINT('Ctrl Pts',(0.533674141594226,-0.0742967091364493,
-0.868149331745851));
#11023=CARTESIAN_POINT('Ctrl Pts',(0.54708917182331,-0.115492077056649,
-0.85981294420286));
#11024=CARTESIAN_POINT('Ctrl Pts',(0.560922177770136,-0.141695629206859,
-0.850993704737257));
#11025=CARTESIAN_POINT('Ctrl Pts',(0.590422647829571,-0.181890537957859,
-0.830754510485543));
#11026=CARTESIAN_POINT('Ctrl Pts',(0.609616703125488,-0.201072148666545,
-0.816896541396381));
#11027=CARTESIAN_POINT('Ctrl Pts',(0.641117951819998,-0.223955109275652,
-0.792310597819928));
#11028=CARTESIAN_POINT('Ctrl Pts',(0.657208095763053,-0.232742381310829,
-0.779109323683612));
#11029=CARTESIAN_POINT('Ctrl Pts',(0.68964083160521,-0.244234834628584,
-0.750552691816206));
#11030=CARTESIAN_POINT('Ctrl Pts',(0.705971972091755,-0.246942143572133,
-0.735185187071673));
#11031=CARTESIAN_POINT('Ctrl Pts',(0.735185187071673,-0.246942143572133,
-0.705971972091754));
#11032=CARTESIAN_POINT('Ctrl Pts',(0.750552691816206,-0.244234834628584,
-0.68964083160521));
#11033=CARTESIAN_POINT('Ctrl Pts',(0.779109323683612,-0.232742381310829,
-0.657208095763053));
#11034=CARTESIAN_POINT('Ctrl Pts',(0.792310597819928,-0.223955109275652,
-0.641117951819998));
#11035=CARTESIAN_POINT('Ctrl Pts',(0.816896541396381,-0.201072148666545,
-0.609616703125488));
#11036=CARTESIAN_POINT('Ctrl Pts',(0.830754510485543,-0.181890537957859,
-0.590422647829571));
#11037=CARTESIAN_POINT('Ctrl Pts',(0.850993704737257,-0.141695629206859,
-0.560922177770136));
#11038=CARTESIAN_POINT('Ctrl Pts',(0.85981294420286,-0.115492077056649,
-0.54708917182331));
#11039=CARTESIAN_POINT('Ctrl Pts',(0.868149331745851,-0.0742967091364493,
-0.533674141594226));
#11040=CARTESIAN_POINT('Ctrl Pts',(0.870146645090731,-0.0609922781173484,
-0.530395067942936));
#11041=CARTESIAN_POINT('Ctrl Pts',(0.871530771444223,-0.0476300000000001,
-0.528110872004958));
#11042=CARTESIAN_POINT('',(0.989696097314,-0.04763,-0.242834539687906));
#11043=CARTESIAN_POINT('Origin',(0.,-0.04763,0.));
#11044=CARTESIAN_POINT('',(0.989696097314,-0.04763,0.242834539687906));
#11045=CARTESIAN_POINT('Ctrl Pts',(0.989696097314,-0.04763,-0.242834539687907));
#11046=CARTESIAN_POINT('Ctrl Pts',(0.990332542620729,-0.0609922781173483,
-0.24024064412003));
#11047=CARTESIAN_POINT('Ctrl Pts',(0.991238884025248,-0.0742967091364493,
-0.236509675094874));
#11048=CARTESIAN_POINT('Ctrl Pts',(0.994830026707808,-0.115492077056649,
-0.221129100087819));
#11049=CARTESIAN_POINT('Ctrl Pts',(0.998375294985966,-0.141695629206859,
-0.205111543747588));
#11050=CARTESIAN_POINT('Ctrl Pts',(1.00492400591205,-0.181890537957859,
-0.169940289819232));
#11051=CARTESIAN_POINT('Ctrl Pts',(1.00869718865384,-0.201072148666545,
-0.1465689792446));
#11052=CARTESIAN_POINT('Ctrl Pts',(1.01358704779679,-0.223955109275652,
-0.106909345252087));
#11053=CARTESIAN_POINT('Ctrl Pts',(1.0156297872271,-0.232742381310829,-0.0861971848975942));
#11054=CARTESIAN_POINT('Ctrl Pts',(1.01837060663223,-0.244234834628584,
-0.0430711894098823));
#11055=CARTESIAN_POINT('Ctrl Pts',(1.019052,-0.246942143572133,-0.0206568624125607));
#11056=CARTESIAN_POINT('Ctrl Pts',(1.019052,-0.246942143572133,0.0206568624125607));
#11057=CARTESIAN_POINT('Ctrl Pts',(1.01837060663223,-0.244234834628584,
0.0430711894098823));
#11058=CARTESIAN_POINT('Ctrl Pts',(1.0156297872271,-0.232742381310829,0.0861971848975942));
#11059=CARTESIAN_POINT('Ctrl Pts',(1.01358704779679,-0.223955109275652,
0.106909345252087));
#11060=CARTESIAN_POINT('Ctrl Pts',(1.00869718865384,-0.201072148666545,
0.1465689792446));
#11061=CARTESIAN_POINT('Ctrl Pts',(1.00492400591205,-0.181890537957859,
0.169940289819232));
#11062=CARTESIAN_POINT('Ctrl Pts',(0.998375294985966,-0.141695629206859,
0.205111543747588));
#11063=CARTESIAN_POINT('Ctrl Pts',(0.994830026707808,-0.115492077056649,
0.221129100087819));
#11064=CARTESIAN_POINT('Ctrl Pts',(0.991238884025248,-0.0742967091364492,
0.236509675094874));
#11065=CARTESIAN_POINT('Ctrl Pts',(0.990332542620729,-0.0609922781173483,
0.24024064412003));
#11066=CARTESIAN_POINT('Ctrl Pts',(0.989696097314,-0.04763,0.242834539687907));
#11067=CARTESIAN_POINT('Origin',(0.,-0.04763,0.));
#11068=CARTESIAN_POINT('Origin',(0.,-0.04763,0.));
#11069=CARTESIAN_POINT('',(0.238183666596899,-0.04763,0.951592097314));
#11070=CARTESIAN_POINT('Origin',(0.,-0.04763,0.));
#11071=CARTESIAN_POINT('Origin',(-1.94289029309402E-16,-0.04763,1.));
#11072=CARTESIAN_POINT('Origin',(-1.94289029309402E-16,0.,1.));
#11073=CARTESIAN_POINT('',(-0.2381836665969,-0.04763,0.951592097314));
#11074=CARTESIAN_POINT('Ctrl Pts',(-0.238183666596899,-0.0476299999999999,
0.951592097314));
#11075=CARTESIAN_POINT('Ctrl Pts',(-0.233157223576062,-0.0740444353928835,
0.952850216871763));
#11076=CARTESIAN_POINT('Ctrl Pts',(-0.223801617934946,-0.0999305678883309,
0.955173119738174));
#11077=CARTESIAN_POINT('Ctrl Pts',(-0.199966927975188,-0.142345102874864,
0.960411259488514));
#11078=CARTESIAN_POINT('Ctrl Pts',(-0.1868781821531,-0.159766064500479,
0.963103647174702));
#11079=CARTESIAN_POINT('Ctrl Pts',(-0.15681442133453,-0.190326085855194,
0.968453058988463));
#11080=CARTESIAN_POINT('Ctrl Pts',(-0.139836317888043,-0.203463743702801,
0.971100730005489));
#11081=CARTESIAN_POINT('Ctrl Pts',(-0.104422493053067,-0.224161999508995,
0.975530745318961));
#11082=CARTESIAN_POINT('Ctrl Pts',(-0.0842175114474176,-0.232861760990032,
0.977553872336861));
#11083=CARTESIAN_POINT('Ctrl Pts',(-0.0421062857595701,-0.244251601209411,
0.980270995488453));
#11084=CARTESIAN_POINT('Ctrl Pts',(-0.0201990724523197,-0.246942143572133,
0.980948));
#11085=CARTESIAN_POINT('Ctrl Pts',(0.020199072452319,-0.246942143572133,
0.980948));
#11086=CARTESIAN_POINT('Ctrl Pts',(0.0421062857595694,-0.244251601209411,
0.980270995488454));
#11087=CARTESIAN_POINT('Ctrl Pts',(0.0842175114474169,-0.232861760990032,
0.977553872336861));
#11088=CARTESIAN_POINT('Ctrl Pts',(0.104422493053067,-0.224161999508995,
0.975530745318961));
#11089=CARTESIAN_POINT('Ctrl Pts',(0.139836317888042,-0.203463743702801,
0.971100730005489));
#11090=CARTESIAN_POINT('Ctrl Pts',(0.15681442133453,-0.190326085855194,
0.968453058988463));
#11091=CARTESIAN_POINT('Ctrl Pts',(0.1868781821531,-0.15976606450048,0.963103647174702));
#11092=CARTESIAN_POINT('Ctrl Pts',(0.199966927975188,-0.142345102874864,
0.960411259488514));
#11093=CARTESIAN_POINT('Ctrl Pts',(0.223801617934945,-0.0999305678883309,
0.955173119738174));
#11094=CARTESIAN_POINT('Ctrl Pts',(0.233157223576061,-0.0740444353928835,
0.952850216871763));
#11095=CARTESIAN_POINT('Ctrl Pts',(0.238183666596899,-0.0476299999999999,
0.951592097314));
#11096=CARTESIAN_POINT('Origin',(-1.94289029309402E-16,-0.04763,1.));
#11097=CARTESIAN_POINT('Origin',(0.,-0.04763,0.));
#11098=CARTESIAN_POINT('',(-0.504455939115715,-0.04763,0.841298510752802));
#11099=CARTESIAN_POINT('Origin',(0.,-0.04763,0.));
#11100=CARTESIAN_POINT('Origin',(-0.707106781186548,-0.04763,0.707106781186547));
#11101=CARTESIAN_POINT('Origin',(-0.707106781186548,0.,0.707106781186547));
#11102=CARTESIAN_POINT('',(-0.841298510752802,-0.04763,0.504455939115715));
#11103=CARTESIAN_POINT('Ctrl Pts',(-0.841298510752802,-0.04763,0.504455939115715));
#11104=CARTESIAN_POINT('Ctrl Pts',(-0.838633903678357,-0.0740444353928835,
0.508899795931835));
#11105=CARTESIAN_POINT('Ctrl Pts',(-0.833661031856294,-0.0999305678883309,
0.517157748491652));
#11106=CARTESIAN_POINT('Ctrl Pts',(-0.820511285096538,-0.142345102874864,
0.537715343527944));
#11107=CARTESIAN_POINT('Ctrl Pts',(-0.813159949759,-0.159766064500479,0.548874290046456));
#11108=CARTESIAN_POINT('Ctrl Pts',(-0.795684265985089,-0.190326085855194,
0.573915184558107));
#11109=CARTESIAN_POINT('Ctrl Pts',(-0.78555112003688,-0.203463743702801,
0.587792702767295));
#11110=CARTESIAN_POINT('Ctrl Pts',(-0.763642258217233,-0.224161999508995,
0.615966552324775));
#11111=CARTESIAN_POINT('Ctrl Pts',(-0.750785745543687,-0.232861760990032,
0.631684198665438));
#11112=CARTESIAN_POINT('Ctrl Pts',(-0.722929908501543,-0.244251601209411,
0.663382628119203));
#11113=CARTESIAN_POINT('Ctrl Pts',(-0.707917883896095,-0.246942143572133,
0.679352081686668));
#11114=CARTESIAN_POINT('Ctrl Pts',(-0.679352081686668,-0.246942143572133,
0.707917883896095));
#11115=CARTESIAN_POINT('Ctrl Pts',(-0.663382628119203,-0.244251601209411,
0.722929908501544));
#11116=CARTESIAN_POINT('Ctrl Pts',(-0.631684198665438,-0.232861760990031,
0.750785745543687));
#11117=CARTESIAN_POINT('Ctrl Pts',(-0.615966552324775,-0.224161999508995,
0.763642258217233));
#11118=CARTESIAN_POINT('Ctrl Pts',(-0.587792702767295,-0.203463743702801,
0.78555112003688));
#11119=CARTESIAN_POINT('Ctrl Pts',(-0.573915184558107,-0.190326085855194,
0.795684265985088));
#11120=CARTESIAN_POINT('Ctrl Pts',(-0.548874290046456,-0.159766064500479,
0.813159949759));
#11121=CARTESIAN_POINT('Ctrl Pts',(-0.537715343527944,-0.142345102874864,
0.820511285096538));
#11122=CARTESIAN_POINT('Ctrl Pts',(-0.517157748491652,-0.0999305678883309,
0.833661031856294));
#11123=CARTESIAN_POINT('Ctrl Pts',(-0.508899795931835,-0.0740444353928835,
0.838633903678357));
#11124=CARTESIAN_POINT('Ctrl Pts',(-0.504455939115716,-0.04763,0.841298510752801));
#11125=CARTESIAN_POINT('Origin',(-0.707106781186548,-0.04763,0.707106781186547));
#11126=CARTESIAN_POINT('Origin',(0.,-0.04763,0.));
#11127=CARTESIAN_POINT('',(-0.951592097314,-0.04763,0.238183666596899));
#11128=CARTESIAN_POINT('Origin',(0.,-0.04763,0.));
#11129=CARTESIAN_POINT('Origin',(-1.,-0.04763,-1.11022302462516E-16));
#11130=CARTESIAN_POINT('Origin',(-1.,0.,-1.11022302462516E-16));
#11131=CARTESIAN_POINT('',(-0.951592097314,-0.04763,-0.2381836665969));
#11132=CARTESIAN_POINT('',(-0.980948,-0.246942143572133,1.08514323328844E-18));
#11133=CARTESIAN_POINT('Ctrl Pts',(-0.951592097314,-0.04763,-0.238183666596899));
#11134=CARTESIAN_POINT('Ctrl Pts',(-0.952850216871763,-0.0740444353928835,
-0.233157223576062));
#11135=CARTESIAN_POINT('Ctrl Pts',(-0.955173119738174,-0.0999305678883309,
-0.223801617934946));
#11136=CARTESIAN_POINT('Ctrl Pts',(-0.960411259488514,-0.142345102874864,
-0.199966927975188));
#11137=CARTESIAN_POINT('Ctrl Pts',(-0.963103647174702,-0.159766064500479,
-0.1868781821531));
#11138=CARTESIAN_POINT('Ctrl Pts',(-0.968453058988463,-0.190326085855194,
-0.15681442133453));
#11139=CARTESIAN_POINT('Ctrl Pts',(-0.971100730005489,-0.203463743702801,
-0.139836317888043));
#11140=CARTESIAN_POINT('Ctrl Pts',(-0.975530745318961,-0.224161999508995,
-0.104422493053067));
#11141=CARTESIAN_POINT('Ctrl Pts',(-0.977553872336861,-0.232861760990032,
-0.0842175114474175));
#11142=CARTESIAN_POINT('Ctrl Pts',(-0.980270995488453,-0.244251601209411,
-0.0421062857595699));
#11143=CARTESIAN_POINT('Ctrl Pts',(-0.980948,-0.246942143572133,-0.0201990724523195));
#11144=CARTESIAN_POINT('Ctrl Pts',(-0.980948,-0.246942143572133,-1.17961196366423E-16));
#11145=CARTESIAN_POINT('Origin',(-1.,-0.04763,-1.11022302462516E-16));
#11146=CARTESIAN_POINT('Ctrl Pts',(-0.980948,-0.246942143572133,-1.17961196366423E-16));
#11147=CARTESIAN_POINT('Ctrl Pts',(-0.980948,-0.246942143572133,0.0201990724523192));
#11148=CARTESIAN_POINT('Ctrl Pts',(-0.980270995488453,-0.244251601209411,
0.0421062857595695));
#11149=CARTESIAN_POINT('Ctrl Pts',(-0.977553872336861,-0.232861760990032,
0.0842175114474169));
#11150=CARTESIAN_POINT('Ctrl Pts',(-0.975530745318961,-0.224161999508995,
0.104422493053066));
#11151=CARTESIAN_POINT('Ctrl Pts',(-0.971100730005489,-0.203463743702801,
0.139836317888042));
#11152=CARTESIAN_POINT('Ctrl Pts',(-0.968453058988463,-0.190326085855194,
0.15681442133453));
#11153=CARTESIAN_POINT('Ctrl Pts',(-0.963103647174702,-0.15976606450048,
0.1868781821531));
#11154=CARTESIAN_POINT('Ctrl Pts',(-0.960411259488514,-0.142345102874864,
0.199966927975188));
#11155=CARTESIAN_POINT('Ctrl Pts',(-0.955173119738174,-0.099930567888331,
0.223801617934945));
#11156=CARTESIAN_POINT('Ctrl Pts',(-0.952850216871763,-0.0740444353928835,
0.233157223576061));
#11157=CARTESIAN_POINT('Ctrl Pts',(-0.951592097314,-0.04763,0.238183666596899));
#11158=CARTESIAN_POINT('Origin',(0.,-0.04763,0.));
#11159=CARTESIAN_POINT('',(-0.841298510752802,-0.04763,-0.504455939115715));
#11160=CARTESIAN_POINT('Origin',(0.,-0.04763,0.));
#11161=CARTESIAN_POINT('Origin',(-0.707106781186547,-0.04763,-0.707106781186548));
#11162=CARTESIAN_POINT('Origin',(-0.707106781186547,0.,-0.707106781186548));
#11163=CARTESIAN_POINT('',(-0.504455939115715,-0.04763,-0.841298510752802));
#11164=CARTESIAN_POINT('Ctrl Pts',(-0.504455939115715,-0.04763,-0.841298510752802));
#11165=CARTESIAN_POINT('Ctrl Pts',(-0.508899795931835,-0.0740444353928835,
-0.838633903678357));
#11166=CARTESIAN_POINT('Ctrl Pts',(-0.517157748491652,-0.0999305678883309,
-0.833661031856294));
#11167=CARTESIAN_POINT('Ctrl Pts',(-0.537715343527944,-0.142345102874864,
-0.820511285096538));
#11168=CARTESIAN_POINT('Ctrl Pts',(-0.548874290046456,-0.159766064500479,
-0.813159949759));
#11169=CARTESIAN_POINT('Ctrl Pts',(-0.573915184558107,-0.190326085855194,
-0.795684265985089));
#11170=CARTESIAN_POINT('Ctrl Pts',(-0.587792702767295,-0.203463743702801,
-0.78555112003688));
#11171=CARTESIAN_POINT('Ctrl Pts',(-0.615966552324775,-0.224161999508995,
-0.763642258217233));
#11172=CARTESIAN_POINT('Ctrl Pts',(-0.631684198665438,-0.232861760990032,
-0.750785745543687));
#11173=CARTESIAN_POINT('Ctrl Pts',(-0.663382628119203,-0.244251601209411,
-0.722929908501543));
#11174=CARTESIAN_POINT('Ctrl Pts',(-0.679352081686668,-0.246942143572133,
-0.707917883896095));
#11175=CARTESIAN_POINT('Ctrl Pts',(-0.707917883896095,-0.246942143572133,
-0.679352081686668));
#11176=CARTESIAN_POINT('Ctrl Pts',(-0.722929908501543,-0.244251601209411,
-0.663382628119203));
#11177=CARTESIAN_POINT('Ctrl Pts',(-0.750785745543687,-0.232861760990032,
-0.631684198665439));
#11178=CARTESIAN_POINT('Ctrl Pts',(-0.763642258217232,-0.224161999508995,
-0.615966552324775));
#11179=CARTESIAN_POINT('Ctrl Pts',(-0.78555112003688,-0.203463743702801,
-0.587792702767295));
#11180=CARTESIAN_POINT('Ctrl Pts',(-0.795684265985088,-0.190326085855194,
-0.573915184558107));
#11181=CARTESIAN_POINT('Ctrl Pts',(-0.813159949759,-0.15976606450048,-0.548874290046456));
#11182=CARTESIAN_POINT('Ctrl Pts',(-0.820511285096538,-0.142345102874864,
-0.537715343527944));
#11183=CARTESIAN_POINT('Ctrl Pts',(-0.833661031856294,-0.0999305678883311,
-0.517157748491652));
#11184=CARTESIAN_POINT('Ctrl Pts',(-0.838633903678357,-0.0740444353928836,
-0.508899795931835));
#11185=CARTESIAN_POINT('Ctrl Pts',(-0.841298510752801,-0.04763,-0.504455939115715));
#11186=CARTESIAN_POINT('Origin',(-0.707106781186547,-0.04763,-0.707106781186548));
#11187=CARTESIAN_POINT('Origin',(0.,-0.04763,0.));
#11188=CARTESIAN_POINT('',(-0.238183666596899,-0.04763,-0.951592097314));
#11189=CARTESIAN_POINT('Origin',(0.,-0.04763,0.));
#11190=CARTESIAN_POINT('Origin',(5.55111512312578E-17,-0.04763,-1.));
#11191=CARTESIAN_POINT('Origin',(5.55111512312578E-17,0.,-1.));
#11192=CARTESIAN_POINT('',(0.238183666596899,-0.04763,-0.951592097314));
#11193=CARTESIAN_POINT('Ctrl Pts',(0.238183666596899,-0.04763,-0.951592097314));
#11194=CARTESIAN_POINT('Ctrl Pts',(0.233157223576062,-0.0740444353928835,
-0.952850216871763));
#11195=CARTESIAN_POINT('Ctrl Pts',(0.223801617934946,-0.099930567888331,
-0.955173119738174));
#11196=CARTESIAN_POINT('Ctrl Pts',(0.199966927975188,-0.142345102874864,
-0.960411259488514));
#11197=CARTESIAN_POINT('Ctrl Pts',(0.1868781821531,-0.15976606450048,-0.963103647174702));
#11198=CARTESIAN_POINT('Ctrl Pts',(0.15681442133453,-0.190326085855194,
-0.968453058988463));
#11199=CARTESIAN_POINT('Ctrl Pts',(0.139836317888042,-0.203463743702801,
-0.971100730005489));
#11200=CARTESIAN_POINT('Ctrl Pts',(0.104422493053067,-0.224161999508995,
-0.975530745318961));
#11201=CARTESIAN_POINT('Ctrl Pts',(0.0842175114474173,-0.232861760990032,
-0.977553872336861));
#11202=CARTESIAN_POINT('Ctrl Pts',(0.0421062857595698,-0.244251601209411,
-0.980270995488453));
#11203=CARTESIAN_POINT('Ctrl Pts',(0.0201990724523194,-0.246942143572133,
-0.980948));
#11204=CARTESIAN_POINT('Ctrl Pts',(-0.0201990724523193,-0.246942143572133,
-0.980948));
#11205=CARTESIAN_POINT('Ctrl Pts',(-0.0421062857595697,-0.244251601209411,
-0.980270995488453));
#11206=CARTESIAN_POINT('Ctrl Pts',(-0.0842175114474171,-0.232861760990032,
-0.977553872336861));
#11207=CARTESIAN_POINT('Ctrl Pts',(-0.104422493053067,-0.224161999508995,
-0.975530745318961));
#11208=CARTESIAN_POINT('Ctrl Pts',(-0.139836317888042,-0.203463743702801,
-0.971100730005489));
#11209=CARTESIAN_POINT('Ctrl Pts',(-0.15681442133453,-0.190326085855194,
-0.968453058988463));
#11210=CARTESIAN_POINT('Ctrl Pts',(-0.1868781821531,-0.15976606450048,-0.963103647174702));
#11211=CARTESIAN_POINT('Ctrl Pts',(-0.199966927975188,-0.142345102874864,
-0.960411259488514));
#11212=CARTESIAN_POINT('Ctrl Pts',(-0.223801617934945,-0.099930567888331,
-0.955173119738174));
#11213=CARTESIAN_POINT('Ctrl Pts',(-0.233157223576062,-0.0740444353928835,
-0.952850216871763));
#11214=CARTESIAN_POINT('Ctrl Pts',(-0.238183666596899,-0.0476299999999999,
-0.951592097314));
#11215=CARTESIAN_POINT('Origin',(5.55111512312578E-17,-0.04763,-1.));
#11216=CARTESIAN_POINT('Origin',(0.,-0.04763,0.));
#11217=CARTESIAN_POINT('',(0.504455939115715,-0.04763,-0.841298510752802));
#11218=CARTESIAN_POINT('Origin',(0.,-0.04763,0.));
#11219=CARTESIAN_POINT('Origin',(0.707106781186548,-0.04763,-0.707106781186547));
#11220=CARTESIAN_POINT('Origin',(0.707106781186548,0.,-0.707106781186547));
#11221=CARTESIAN_POINT('',(0.841298510752802,-0.04763,-0.504455939115715));
#11222=CARTESIAN_POINT('Ctrl Pts',(0.841298510752802,-0.04763,-0.504455939115715));
#11223=CARTESIAN_POINT('Ctrl Pts',(0.838633903678357,-0.0740444353928835,
-0.508899795931835));
#11224=CARTESIAN_POINT('Ctrl Pts',(0.833661031856294,-0.0999305678883309,
-0.517157748491652));
#11225=CARTESIAN_POINT('Ctrl Pts',(0.820511285096538,-0.142345102874864,
-0.537715343527944));
#11226=CARTESIAN_POINT('Ctrl Pts',(0.813159949759,-0.159766064500479,-0.548874290046456));
#11227=CARTESIAN_POINT('Ctrl Pts',(0.795684265985088,-0.190326085855194,
-0.573915184558107));
#11228=CARTESIAN_POINT('Ctrl Pts',(0.78555112003688,-0.203463743702801,
-0.587792702767295));
#11229=CARTESIAN_POINT('Ctrl Pts',(0.763642258217233,-0.224161999508995,
-0.615966552324775));
#11230=CARTESIAN_POINT('Ctrl Pts',(0.750785745543687,-0.232861760990032,
-0.631684198665438));
#11231=CARTESIAN_POINT('Ctrl Pts',(0.722929908501543,-0.244251601209411,
-0.663382628119203));
#11232=CARTESIAN_POINT('Ctrl Pts',(0.707917883896095,-0.246942143572133,
-0.679352081686668));
#11233=CARTESIAN_POINT('Ctrl Pts',(0.679352081686668,-0.246942143572133,
-0.707917883896095));
#11234=CARTESIAN_POINT('Ctrl Pts',(0.663382628119203,-0.244251601209411,
-0.722929908501543));
#11235=CARTESIAN_POINT('Ctrl Pts',(0.631684198665438,-0.232861760990032,
-0.750785745543687));
#11236=CARTESIAN_POINT('Ctrl Pts',(0.615966552324775,-0.224161999508995,
-0.763642258217232));
#11237=CARTESIAN_POINT('Ctrl Pts',(0.587792702767295,-0.203463743702801,
-0.78555112003688));
#11238=CARTESIAN_POINT('Ctrl Pts',(0.573915184558107,-0.190326085855194,
-0.795684265985088));
#11239=CARTESIAN_POINT('Ctrl Pts',(0.548874290046456,-0.159766064500479,
-0.813159949759));
#11240=CARTESIAN_POINT('Ctrl Pts',(0.537715343527944,-0.142345102874864,
-0.820511285096538));
#11241=CARTESIAN_POINT('Ctrl Pts',(0.517157748491652,-0.099930567888331,
-0.833661031856294));
#11242=CARTESIAN_POINT('Ctrl Pts',(0.508899795931835,-0.0740444353928835,
-0.838633903678357));
#11243=CARTESIAN_POINT('Ctrl Pts',(0.504455939115715,-0.04763,-0.841298510752801));
#11244=CARTESIAN_POINT('Origin',(0.707106781186548,-0.04763,-0.707106781186547));
#11245=CARTESIAN_POINT('Origin',(0.,-0.166705,0.));
#11246=CARTESIAN_POINT('',(-0.980948,-0.28578,1.20131482833E-16));
#11247=CARTESIAN_POINT('Origin',(0.,-0.28578,0.));
#11248=CARTESIAN_POINT('',(-0.980948,-0.166705,1.20131482833E-16));
#11249=CARTESIAN_POINT('',(0.951592097314,-0.04763,0.238183666596899));
#11250=CARTESIAN_POINT('Origin',(0.,-0.04763,0.));
#11251=CARTESIAN_POINT('',(0.951592097314,-0.04763,-0.238183666596899));
#11252=CARTESIAN_POINT('Ctrl Pts',(0.951592097314,-0.04763,0.238183666596899));
#11253=CARTESIAN_POINT('Ctrl Pts',(0.952850216871763,-0.0740444353928835,
0.233157223576062));
#11254=CARTESIAN_POINT('Ctrl Pts',(0.955173119738174,-0.099930567888331,
0.223801617934945));
#11255=CARTESIAN_POINT('Ctrl Pts',(0.960411259488514,-0.142345102874864,
0.199966927975188));
#11256=CARTESIAN_POINT('Ctrl Pts',(0.963103647174702,-0.15976606450048,
0.1868781821531));
#11257=CARTESIAN_POINT('Ctrl Pts',(0.968453058988463,-0.190326085855194,
0.15681442133453));
#11258=CARTESIAN_POINT('Ctrl Pts',(0.971100730005489,-0.203463743702801,
0.139836317888042));
#11259=CARTESIAN_POINT('Ctrl Pts',(0.975530745318961,-0.224161999508995,
0.104422493053067));
#11260=CARTESIAN_POINT('Ctrl Pts',(0.977553872336861,-0.232861760990032,
0.0842175114474172));
#11261=CARTESIAN_POINT('Ctrl Pts',(0.980270995488453,-0.244251601209411,
0.0421062857595697));
#11262=CARTESIAN_POINT('Ctrl Pts',(0.980948,-0.246942143572133,0.0201990724523194));
#11263=CARTESIAN_POINT('Ctrl Pts',(0.980948,-0.246942143572133,-0.0201990724523194));
#11264=CARTESIAN_POINT('Ctrl Pts',(0.980270995488453,-0.244251601209411,
-0.0421062857595697));
#11265=CARTESIAN_POINT('Ctrl Pts',(0.977553872336861,-0.232861760990032,
-0.0842175114474172));
#11266=CARTESIAN_POINT('Ctrl Pts',(0.975530745318961,-0.224161999508995,
-0.104422493053067));
#11267=CARTESIAN_POINT('Ctrl Pts',(0.971100730005489,-0.203463743702801,
-0.139836317888042));
#11268=CARTESIAN_POINT('Ctrl Pts',(0.968453058988463,-0.190326085855194,
-0.15681442133453));
#11269=CARTESIAN_POINT('Ctrl Pts',(0.963103647174702,-0.15976606450048,
-0.1868781821531));
#11270=CARTESIAN_POINT('Ctrl Pts',(0.960411259488514,-0.142345102874864,
-0.199966927975188));
#11271=CARTESIAN_POINT('Ctrl Pts',(0.955173119738174,-0.099930567888331,
-0.223801617934945));
#11272=CARTESIAN_POINT('Ctrl Pts',(0.952850216871763,-0.0740444353928835,
-0.233157223576062));
#11273=CARTESIAN_POINT('Ctrl Pts',(0.951592097314,-0.0476299999999999,-0.238183666596899));
#11274=CARTESIAN_POINT('Origin',(0.,-0.04763,0.));
#11275=CARTESIAN_POINT('Origin',(0.,-0.04763,0.));
#11276=CARTESIAN_POINT('Origin',(1.,-0.04763,0.));
#11277=CARTESIAN_POINT('Origin',(1.,0.,0.));
#11278=CARTESIAN_POINT('Origin',(1.,-0.04763,0.));
#11279=CARTESIAN_POINT('Origin',(0.,-0.28578,0.));
#11280=CARTESIAN_POINT('Origin',(0.,-0.04763,0.));
#12340=UNCERTAINTY_MEASURE_WITH_UNIT(LENGTH_MEASURE(0.001),#12414,
'DISTANCE_ACCURACY_VALUE',
'Maximum model space distance between geometric entities at asserted c
onnectivities');
#12367=UNCERTAINTY_MEASURE_WITH_UNIT(LENGTH_MEASURE(0.001),#12414,
'DISTANCE_ACCURACY_VALUE',
'Maximum model space distance between geometric entities at asserted c
onnectivities');
#12386=(
GEOMETRIC_REPRESENTATION_CONTEXT(3)
GLOBAL_UNCERTAINTY_ASSIGNED_CONTEXT((#12340))
GLOBAL_UNIT_ASSIGNED_CONTEXT((#12414,#12416,#12417))
REPRESENTATION_CONTEXT('','3D')
);
#12413=(
GEOMETRIC_REPRESENTATION_CONTEXT(3)
GLOBAL_UNCERTAINTY_ASSIGNED_CONTEXT((#12367))
GLOBAL_UNIT_ASSIGNED_CONTEXT((#12414,#12416,#12417))
REPRESENTATION_CONTEXT('','3D')
);
#12414=(
LENGTH_UNIT()
NAMED_UNIT(*)
SI_UNIT(.CENTI.,.METRE.)
);
#12416=(
NAMED_UNIT(*)
PLANE_ANGLE_UNIT()
SI_UNIT($,.RADIAN.)
);
#12417=(
NAMED_UNIT(*)
SI_UNIT($,.STERADIAN.)
SOLID_ANGLE_UNIT()
);
#12436=SHAPE_DEFINITION_REPRESENTATION(#12481,#12589);
#12481=PRODUCT_DEFINITION_SHAPE('',$,#12635);
#12589=SHAPE_REPRESENTATION('',(#7385),#12386);
#12616=PRODUCT_DEFINITION_CONTEXT('part definition',#12753,'design');
#12635=PRODUCT_DEFINITION('Cage','Cage',#12680,#12616);
#12680=PRODUCT_DEFINITION_FORMATION('',$,#12773);
#12753=APPLICATION_CONTEXT(
'Core Data for Automotive Mechanical Design Process');
#12754=PRODUCT_CONTEXT('part definition',#12753,'mechanical');
#12773=PRODUCT('Cage','Cage','Cage',(#12754));
#12863=COLOUR_RGB('Grey',0.48,0.52,0.57);
#12864=FILL_AREA_STYLE_COLOUR('',#12863);
#12865=FILL_AREA_STYLE('',(#12864));
#12866=SURFACE_STYLE_FILL_AREA(#12865);
#12867=SURFACE_SIDE_STYLE('',(#12866));
#12868=SURFACE_STYLE_USAGE(.BOTH.,#12867);
#12869=PRESENTATION_STYLE_ASSIGNMENT((#12868));
ENDSEC;
END-ISO-10303-21;
